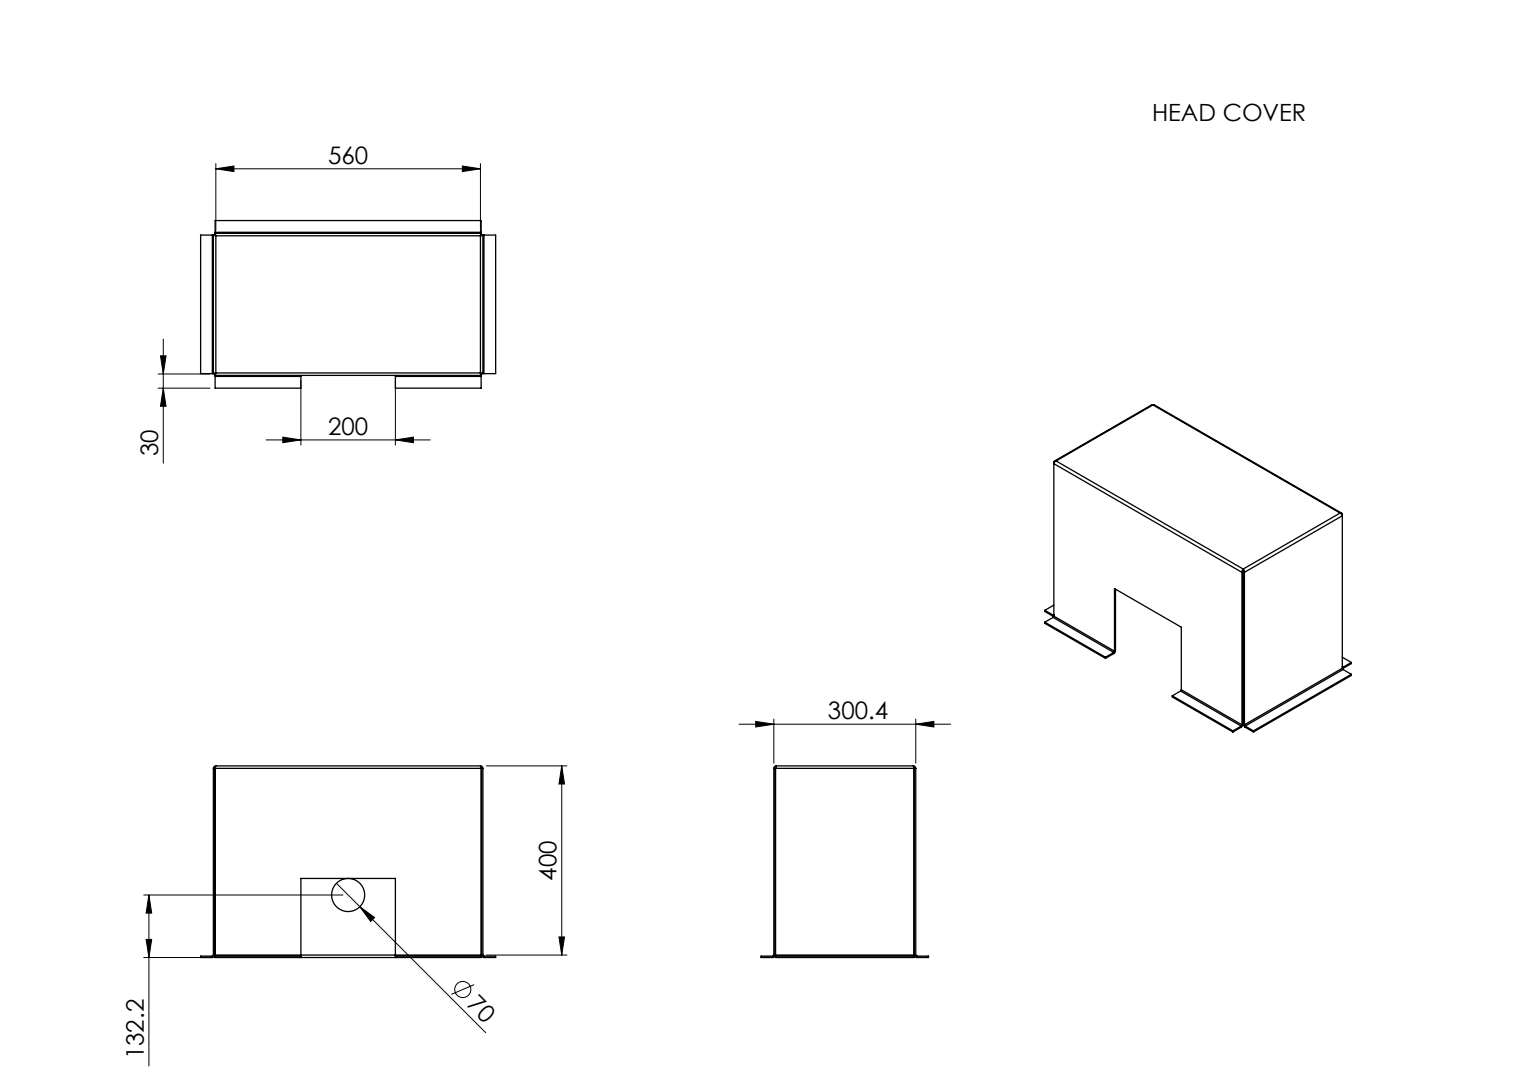
ISO-10303-21;
HEADER;
FILE_DESCRIPTION (('STEP AP214'),
    '1' );
FILE_NAME ('head cover.step',
    '2026-10-31T03:46:07',
    ( '' ),
    ( '' ),
    'SwSTEP 2.0',
    'SolidWorks 2026',
    '' );
FILE_SCHEMA (( 'AUTOMOTIVE_DESIGN' ));
ENDSEC;

DATA;
#14=DIRECTION ( 'NONE',  ( 1.000000000000000000, -6.640089860198304064E-16, -0.000000000000000000 ) ) ;
#17=AXIS2_PLACEMENT_3D ( 'NONE', #8698, #6875, #2876 ) ;
#23=DIRECTION ( 'NONE',  ( -0.000000000000000000, -0.000000000000000000, 1.000000000000000000 ) ) ;
#39=VECTOR ( 'NONE', #3560, 1000.000000000000000 ) ;
#44=CARTESIAN_POINT ( 'NONE',  ( 280.4976310729377929, 269.6958543268122526, -146.0927021017107279 ) ) ;
#46=DIRECTION ( 'NONE',  ( 1.000000000000000000, -0.000000000000000000, -0.000000000000000000 ) ) ;
#47=EDGE_LOOP ( 'NONE', ( #6115, #19407 ) ) ;
#50=CARTESIAN_POINT ( 'NONE',  ( 281.4928932188134354, -129.2000000000000455, -150.2000000000013245 ) ) ;
#59=EDGE_CURVE ( 'NONE', #14664, #1301, #12963, .T. ) ;
#62=EDGE_CURVE ( 'NONE', #22159, #2544, #22076, .T. ) ;
#67=VERTEX_POINT ( 'NONE', #12958 ) ;
#68=CARTESIAN_POINT ( 'NONE',  ( 281.3673618604586295, 268.0905802150185195, -147.1999999999998749 ) ) ;
#84=EDGE_CURVE ( 'NONE', #20571, #4595, #14131, .T. ) ;
#87=DIRECTION ( 'NONE',  ( -1.000000000000000000, -0.000000000000000000, -0.000000000000000000 ) ) ;
#101=ORIENTED_EDGE ( 'NONE', *, *, #6605, .F. ) ;
#117=ADVANCED_FACE ( 'NONE', ( #14863 ), #10660, .T. ) ;
#128=CARTESIAN_POINT ( 'NONE',  ( 281.4928932188134354, -132.2000000000000455, -177.2000000000013529 ) ) ;
#129=AXIS2_PLACEMENT_3D ( 'NONE', #9738, #17091, #22629 ) ;
#131=CARTESIAN_POINT ( 'NONE',  ( 284.6730547946947354, 270.1059783239180661, 146.0571358042176087 ) ) ;
#139=FACE_BOUND ( 'NONE', #47, .T. ) ;
#146=ADVANCED_FACE ( 'NONE', ( #21970 ), #14402, .F. ) ;
#147=ORIENTED_EDGE ( 'NONE', *, *, #7523, .T. ) ;
#167=DIRECTION ( 'NONE',  ( 0.000000000000000000, 0.000000000000000000, -1.000000000000000000 ) ) ;
#168=VECTOR ( 'NONE', #12826, 1000.000000000000000 ) ;
#171=EDGE_CURVE ( 'NONE', #22518, #4872, #9420, .T. ) ;
#177=CARTESIAN_POINT ( 'NONE',  ( -34.75000000000005684, 100.0000000000000000, 150.2000000000009550 ) ) ;
#185=EDGE_CURVE ( 'NONE', #19310, #4045, #11744, .T. ) ;
#202=CIRCLE ( 'NONE', #14864, 2.649999999999971934 ) ;
#210=CARTESIAN_POINT ( 'NONE',  ( 281.1021437883072167, 269.7094021484633686, -145.4974534559949859 ) ) ;
#211=EDGE_LOOP ( 'NONE', ( #6410, #3286, #15490, #21044 ) ) ;
#212=ADVANCED_FACE ( 'NONE', ( #22806 ), #18937, .T. ) ;
#225=VECTOR ( 'NONE', #9857, 1000.000000000000000 ) ;
#231=ORIENTED_EDGE ( 'NONE', *, *, #16834, .F. ) ;
#233=LINE ( 'NONE', #3596, #6438 ) ;
#244=DIRECTION ( 'NONE',  ( 1.000000000000000000, -0.000000000000000000, -0.000000000000000000 ) ) ;
#249=CARTESIAN_POINT ( 'NONE',  ( -100.0000000000000000, 35.00000000000009948, 150.2000000000008413 ) ) ;
#263=DIRECTION ( 'NONE',  ( 1.000000000000000000, 0.000000000000000000, 0.000000000000000000 ) ) ;
#264=ORIENTED_EDGE ( 'NONE', *, *, #1576, .T. ) ;
#265=CARTESIAN_POINT ( 'NONE',  ( 280.3431883566700549, 273.0000000000000568, -145.0627246244601167 ) ) ;
#270=ADVANCED_FACE ( 'NONE', ( #15223 ), #15473, .F. ) ;
#276=ORIENTED_EDGE ( 'NONE', *, *, #12482, .T. ) ;
#284=CARTESIAN_POINT ( 'NONE',  ( -280.9952621458755857, 268.9079617568159506, -146.9223300543793584 ) ) ;
#289=LINE ( 'NONE', #9594, #2999 ) ;
#291=AXIS2_PLACEMENT_3D ( 'NONE', #21240, #8314, #10626 ) ;
#292=CARTESIAN_POINT ( 'NONE',  ( 281.8958543268121844, 268.8927021017106540, 145.9952621458756710 ) ) ;
#297=FACE_OUTER_BOUND ( 'NONE', #16595, .T. ) ;
#313=EDGE_CURVE ( 'NONE', #14070, #15403, #21354, .T. ) ;
#331=VECTOR ( 'NONE', #4440, 1000.000000000000000 ) ;
#336=AXIS2_PLACEMENT_3D ( 'NONE', #12749, #1460, #5215 ) ;
#340=DIRECTION ( 'NONE',  ( -1.000000000000000000, -0.000000000000000000, -0.000000000000000000 ) ) ;
#341=AXIS2_PLACEMENT_3D ( 'NONE', #13845, #16102, #21173 ) ;
#351=ADVANCED_FACE ( 'NONE', ( #21114 ), #3118, .F. ) ;
#352=ORIENTED_EDGE ( 'NONE', *, *, #7831, .T. ) ;
#355=AXIS2_PLACEMENT_3D ( 'NONE', #12926, #14588, #3930 ) ;
#367=DIRECTION ( 'NONE',  ( 1.000000000000000000, 0.000000000000000000, -0.000000000000000000 ) ) ;
#368=EDGE_LOOP ( 'NONE', ( #6453, #4293, #7528, #16012 ) ) ;
#372=AXIS2_PLACEMENT_3D ( 'NONE', #12914, #5396, #21586 ) ;
#381=VECTOR ( 'NONE', #12199, 1000.000000000000000 ) ;
#382=CARTESIAN_POINT ( 'NONE',  ( -280.4973317504632746, 272.3135885331259374, -147.6045710003933493 ) ) ;
#384=CARTESIAN_POINT ( 'NONE',  ( -281.4538215477170979, 269.4574776399289249, -145.6842353883612304 ) ) ;
#386=LINE ( 'NONE', #9552, #2401 ) ;
#396=CARTESIAN_POINT ( 'NONE',  ( 280.4976310729377929, 272.3436892194421830, -147.6188186979286456 ) ) ;
#416=CIRCLE ( 'NONE', #20853, 2.649999999999975486 ) ;
#421=CARTESIAN_POINT ( 'NONE',  ( -280.1244266708878854, 270.0000000000000000, -145.2880230824753198 ) ) ;
#430=EDGE_LOOP ( 'NONE', ( #19662, #7339, #6676, #22145 ) ) ;
#458=ADVANCED_FACE ( 'NONE', ( #6629 ), #8833, .F. ) ;
#459=CARTESIAN_POINT ( 'NONE',  ( 282.1854425596106921, 268.0906609804447953, -146.3673129565597719 ) ) ;
#460=EDGE_CURVE ( 'NONE', #4025, #10987, #14591, .T. ) ;
#472=CARTESIAN_POINT ( 'NONE',  ( 281.9223300543793584, 268.9079617568158938, -145.9952621458755857 ) ) ;
#477=ORIENTED_EDGE ( 'NONE', *, *, #2966, .T. ) ;
#478=ORIENTED_EDGE ( 'NONE', *, *, #11288, .T. ) ;
#481=ADVANCED_FACE ( 'NONE', ( #3691 ), #14484, .T. ) ;
#484=EDGE_LOOP ( 'NONE', ( #635, #3339, #8583, #20621 ) ) ;
#497=CARTESIAN_POINT ( 'NONE',  ( -280.1452901038203436, 270.0000000000000000, -145.0627656775836556 ) ) ;
#500=DIRECTION ( 'NONE',  ( 0.000000000000000000, -3.495664435217746987E-15, -1.000000000000000000 ) ) ;
#502=FACE_BOUND ( 'NONE', #1152, .T. ) ;
#503=DIRECTION ( 'NONE',  ( 0.000000000000000000, 0.000000000000000000, 1.000000000000000000 ) ) ;
#505=VECTOR ( 'NONE', #4591, 1000.000000000000000 ) ;
#515=EDGE_CURVE ( 'NONE', #17412, #8986, #3345, .T. ) ;
#530=CARTESIAN_POINT ( 'NONE',  ( -282.0873946496627127, 268.5095819834011763, 146.1815513148989965 ) ) ;
#539=VERTEX_POINT ( 'NONE', #2242 ) ;
#541=CYLINDRICAL_SURFACE ( 'NONE', #20678, 2.199999999999979750 ) ;
#549=CARTESIAN_POINT ( 'NONE',  ( -280.0000000000000568, 272.9999999999999432, 145.0000000000000284 ) ) ;
#558=EDGE_CURVE ( 'NONE', #7386, #12822, #19852, .T. ) ;
#559=CARTESIAN_POINT ( 'NONE',  ( -288.2000000000013529, -89.99999999999897682, 26.98333333333330231 ) ) ;
#577=EDGE_CURVE ( 'NONE', #539, #10685, #15195, .T. ) ;
#584=FACE_BOUND ( 'NONE', #11064, .T. ) ;
#594=EDGE_CURVE ( 'NONE', #15324, #17025, #2363, .T. ) ;
#603=VERTEX_POINT ( 'NONE', #15316 ) ;
#604=CARTESIAN_POINT ( 'NONE',  ( 285.2000000000008981, 9.892604858775018348E-13, 146.4928932188134638 ) ) ;
#614=CARTESIAN_POINT ( 'NONE',  ( 280.6822561791009889, 272.9663407402829876, 145.1247002395580807 ) ) ;
#617=CARTESIAN_POINT ( 'NONE',  ( 40.00000000000000000, 100.0000000000000000, 150.2000000000009550 ) ) ;
#618=ORIENTED_EDGE ( 'NONE', *, *, #2883, .F. ) ;
#621=SURFACE_SIDE_STYLE ('',( #11763 ) ) ;
#625=DIRECTION ( 'NONE',  ( -0.000000000000000000, -0.000000000000000000, 1.000000000000000000 ) ) ;
#631=CARTESIAN_POINT ( 'NONE',  ( 282.6045710003933777, 272.3135885331259942, -145.4973317504631609 ) ) ;
#632=EDGE_LOOP ( 'NONE', ( #21838, #2466, #15904, #21981 ) ) ;
#635=ORIENTED_EDGE ( 'NONE', *, *, #22905, .T. ) ;
#640=VERTEX_POINT ( 'NONE', #19144 ) ;
#641=CARTESIAN_POINT ( 'NONE',  ( -281.3684665762324926, 268.0840560642351988, -147.1696999999999207 ) ) ;
#662=CARTESIAN_POINT ( 'NONE',  ( -285.2000000000013529, -89.99999999999896261, -40.33333333333332860 ) ) ;
#672=PLANE ( 'NONE',  #1139 ) ;
#674=ORIENTED_EDGE ( 'NONE', *, *, #10081, .T. ) ;
#678=AXIS2_PLACEMENT_3D ( 'NONE', #5455, #7253, #20169 ) ;
#686=DIRECTION ( 'NONE',  ( -1.000000000000000000, 3.495664435217746592E-15, -0.000000000000000000 ) ) ;
#689=FACE_OUTER_BOUND ( 'NONE', #8839, .T. ) ;
#693=ORIENTED_EDGE ( 'NONE', *, *, #16007, .T. ) ;
#697=CARTESIAN_POINT ( 'NONE',  ( -282.2000000000006708, 90.00000000000102318, -32.35000000000004405 ) ) ;
#729=FILL_AREA_STYLE ('',( #3980 ) ) ;
#733=VERTEX_POINT ( 'NONE', #21327 ) ;
#734=EDGE_CURVE ( 'NONE', #21032, #15145, #6249, .T. ) ;
#736=CARTESIAN_POINT ( 'NONE',  ( 0.000000000000000000, -132.2000000000000455, 7.703011046602857601E-15 ) ) ;
#746=VECTOR ( 'NONE', #8115, 1000.000000000000000 ) ;
#749=CARTESIAN_POINT ( 'NONE',  ( -280.4976310729379065, 272.3436892194421262, 147.6188186979287025 ) ) ;
#751=ORIENTED_EDGE ( 'NONE', *, *, #3968, .T. ) ;
#752=ADVANCED_FACE ( 'NONE', ( #913 ), #15562, .F. ) ;
#756=DIRECTION ( 'NONE',  ( 1.000000000000000000, 0.000000000000000000, 0.000000000000000000 ) ) ;
#761=CARTESIAN_POINT ( 'NONE',  ( -280.6220388411722411, 271.9822575857424454, -148.2140793454688037 ) ) ;
#769=LINE ( 'NONE', #1117, #4265 ) ;
#770=CARTESIAN_POINT ( 'NONE',  ( 284.1582675804705218, 270.9956429438695409, 145.8708543776411943 ) ) ;
#775=CARTESIAN_POINT ( 'NONE',  ( 45.00000000000000000, 272.9999999999999432, 5.249999999999973355 ) ) ;
#787=EDGE_CURVE ( 'NONE', #23122, #3613, #19452, .T. ) ;
#813=ORIENTED_EDGE ( 'NONE', *, *, #10441, .T. ) ;
#822=DIRECTION ( 'NONE',  ( 0.000000000000000000, -1.000000000000000000, -3.172065784643303781E-15 ) ) ;
#823=CARTESIAN_POINT ( 'NONE',  ( -280.0000000000000568, 272.9999999999999432, 145.0000000000000284 ) ) ;
#830=ORIENTED_EDGE ( 'NONE', *, *, #12374, .F. ) ;
#838=DIRECTION ( 'NONE',  ( 1.000000000000000000, 0.000000000000000000, -0.000000000000000000 ) ) ;
#845=DIRECTION ( 'NONE',  ( 0.000000000000000000, 0.000000000000000000, -1.000000000000000000 ) ) ;
#851=VECTOR ( 'NONE', #20972, 1000.000000000000000 ) ;
#858=CARTESIAN_POINT ( 'NONE',  ( -281.2440776823446527, 269.1689414351989740, 150.0938770989752982 ) ) ;
#861=ADVANCED_FACE ( 'NONE', ( #22030 ), #21930, .F. ) ;
#862=FACE_BOUND ( 'NONE', #14300, .T. ) ;
#872=EDGE_CURVE ( 'NONE', #15992, #2924, #11012, .T. ) ;
#887=ORIENTED_EDGE ( 'NONE', *, *, #20314, .T. ) ;
#899=CARTESIAN_POINT ( 'NONE',  ( 281.7502846751310699, 269.1405375976306686, 145.8716261326570702 ) ) ;
#905=DIRECTION ( 'NONE',  ( 0.000000000000000000, -1.000000000000000000, 0.000000000000000000 ) ) ;
#913=FACE_OUTER_BOUND ( 'NONE', #11726, .T. ) ;
#933=CARTESIAN_POINT ( 'NONE',  ( 280.2481149223240209, 269.9433523009094529, 145.5743436287470161 ) ) ;
#955=PLANE ( 'NONE',  #7810 ) ;
#967=CARTESIAN_POINT ( 'NONE',  ( 281.4928932188133217, -127.0000000000000568, 152.4000000000014268 ) ) ;
#971=CARTESIAN_POINT ( 'NONE',  ( -281.2440776823446527, 268.3758453455903918, 147.1427398886702917 ) ) ;
#988=CARTESIAN_POINT ( 'NONE',  ( -281.4928932188134922, -127.0000000000000568, -150.2000000000013245 ) ) ;
#990=CARTESIAN_POINT ( 'NONE',  ( -281.4928932188135491, -132.2000000000000455, 177.2000000000014097 ) ) ;
#995=EDGE_CURVE ( 'NONE', #20571, #18758, #14923, .T. ) ;
#1006=VECTOR ( 'NONE', #14424, 1000.000000000000000 ) ;
#1011=CARTESIAN_POINT ( 'NONE',  ( -100.0000000000001137, -129.2000000000000455, 7.690461757479017101E-15 ) ) ;
#1020=ORIENTED_EDGE ( 'NONE', *, *, #23692, .T. ) ;
#1021=CARTESIAN_POINT ( 'NONE',  ( 285.2000000000013529, -129.2000000000000455, 146.4928932188134638 ) ) ;
#1030=ADVANCED_FACE ( 'NONE', ( #12132 ), #13818, .F. ) ;
#1049=CARTESIAN_POINT ( 'NONE',  ( -285.1663407402830899, 268.4822561791010571, 146.3681929792554399 ) ) ;
#1055=ORIENTED_EDGE ( 'NONE', *, *, #2680, .T. ) ;
#1058=ORIENTED_EDGE ( 'NONE', *, *, #22905, .F. ) ;
#1075=EDGE_CURVE ( 'NONE', #603, #2349, #20263, .T. ) ;
#1077=CIRCLE ( 'NONE', #20722, 2.649999999999975486 ) ;
#1087=B_SPLINE_CURVE_WITH_KNOTS ( 'NONE', 3,
 ( #11660, #265, #22590, #2179, #6054, #2428, #631, #20787, #11774, #19083, #2552, #18965, #5699, #16697, #13235, #7624, #22361, #15016, #20427, #4250 ),
 .UNSPECIFIED., .F., .F.,
 ( 4, 2, 2, 2, 2, 2, 2, 2, 2, 4 ),
 ( 0.000000000000000000, 0.001035985217005840064, 0.002071970434011680129, 0.003107955651017520193, 0.003625948259520417674, 0.004143940868023315155, 0.005179926085028993023, 0.006215911302034670891, 0.007251896519040349626, 0.008287881736046026626 ),
 .UNSPECIFIED. ) ;
#1093=B_SPLINE_SURFACE_WITH_KNOTS ( 'NONE', 1, 3, ( 
 ( #5953, #2443, #17190, #3899, #761, #22488, #15389, #11788, #13611, #5842 ),
 ( #8012, #9835, #15273, #22379, #13362, #18733, #9472, #5713, #22605, #11672 ),
 ( #9589, #421, #7890, #13250, #20553, #4129, #284, #17313, #15155, #7774 ),
 ( #20804, #4007, #11424, #15036, #20921, #8143, #20674, #2194, #641, #16953 ) ),
 .UNSPECIFIED., .F., .F., .F.,
 ( 2, 1, 1, 2 ),
 ( 4, 2, 2, 2, 4 ),
 ( -0.01000000000000000021, 0.000000000000000000, 1.000000000000000000, 1.010099999999999998 ),
 ( 0.000000000000000000, 0.2500000000000000000, 0.5000000000000000000, 0.7500000000000000000, 1.000000000000000000 ),
 .UNSPECIFIED. ) ;
#1099=ORIENTED_EDGE ( 'NONE', *, *, #23146, .F. ) ;
#1102=CARTESIAN_POINT ( 'NONE',  ( -281.4928932188135491, 267.7999999999999545, 147.1999999999999886 ) ) ;
#1114=VECTOR ( 'NONE', #12180, 1000.000000000000000 ) ;
#1115=VECTOR ( 'NONE', #10599, 1000.000000000000000 ) ;
#1117=CARTESIAN_POINT ( 'NONE',  ( 35.00000000000000711, 0.000000000000000000, -177.2000000000013529 ) ) ;
#1119=AXIS2_PLACEMENT_3D ( 'NONE', #5628, #14944, #12816 ) ;
#1123=DIRECTION ( 'NONE',  ( -0.000000000000000000, 1.000000000000000000, -4.183096374613631247E-18 ) ) ;
#1124=CARTESIAN_POINT ( 'NONE',  ( -285.0646579186753797, 269.1610889986682196, -146.2440776823445390 ) ) ;
#1128=DIRECTION ( 'NONE',  ( -0.000000000000000000, 0.000000000000000000, -1.000000000000000000 ) ) ;
#1130=ADVANCED_FACE ( 'NONE', ( #17882 ), #23560, .F. ) ;
#1139=AXIS2_PLACEMENT_3D ( 'NONE', #8048, #21315, #12297 ) ;
#1147=CARTESIAN_POINT ( 'NONE',  ( 280.9755403010747159, 269.7771302778489826, 145.4357197208657340 ) ) ;
#1152=EDGE_LOOP ( 'NONE', ( #4727, #12791 ) ) ;
#1162=CIRCLE ( 'NONE', #12782, 2.199999999999979750 ) ;
#1164=CARTESIAN_POINT ( 'NONE',  ( -281.4928932188135491, -132.2000000000000455, 150.2000000000013813 ) ) ;
#1167=CARTESIAN_POINT ( 'NONE',  ( -283.7968359015655437, 271.3570580646226631, -145.7774350431394907 ) ) ;
#1174=DIRECTION ( 'NONE',  ( 0.000000000000000000, 0.000000000000000000, 1.000000000000000000 ) ) ;
#1176=DIRECTION ( 'NONE',  ( 4.183096374613631247E-18, -1.000000000000000000, 0.000000000000000000 ) ) ;
#1183=VECTOR ( 'NONE', #18740, 1000.000000000000000 ) ;
#1185=ORIENTED_EDGE ( 'NONE', *, *, #3808, .F. ) ;
#1186=CARTESIAN_POINT ( 'NONE',  ( -281.2431816561011715, 268.3724317483737423, -147.1290760626066856 ) ) ;
#1203=ORIENTED_EDGE ( 'NONE', *, *, #19391, .F. ) ;
#1211=ORIENTED_EDGE ( 'NONE', *, *, #5766, .T. ) ;
#1213=DIRECTION ( 'NONE',  ( -0.000000000000000000, 7.709882115452476934E-17, -1.000000000000000000 ) ) ;
#1216=VERTEX_POINT ( 'NONE', #21849 ) ;
#1221=EDGE_CURVE ( 'NONE', #21906, #11842, #4475, .T. ) ;
#1224=ORIENTED_EDGE ( 'NONE', *, *, #9825, .T. ) ;
#1226=CARTESIAN_POINT ( 'NONE',  ( 0.000000000000000000, 5.173457871231059415E-13, -150.2000000000008981 ) ) ;
#1227=FACE_OUTER_BOUND ( 'NONE', #1740, .T. ) ;
#1238=DIRECTION ( 'NONE',  ( -0.000000000000000000, 0.000000000000000000, 1.000000000000000000 ) ) ;
#1274=CARTESIAN_POINT ( 'NONE',  ( -284.2295083325149108, 270.8299054689546779, -145.9020829022173871 ) ) ;
#1284=VECTOR ( 'NONE', #5986, 1000.000000000000000 ) ;
#1285=CARTESIAN_POINT ( 'NONE',  ( 281.4928932188133786, -129.2000000000000455, 177.2000000000014097 ) ) ;
#1289=DIRECTION ( 'NONE',  ( 4.183096374613631247E-18, 1.000000000000000000, 0.000000000000000000 ) ) ;
#1291=ORIENTED_EDGE ( 'NONE', *, *, #17411, .F. ) ;
#1293=LINE ( 'NONE', #1412, #19171 ) ;
#1301=VERTEX_POINT ( 'NONE', #22323 ) ;
#1303=ADVANCED_FACE ( 'NONE', ( #4461 ), #20888, .F. ) ;
#1308=ORIENTED_EDGE ( 'NONE', *, *, #15523, .F. ) ;
#1320=CARTESIAN_POINT ( 'NONE',  ( -312.2000000000014666, -132.2000000000000455, -146.4928932188134070 ) ) ;
#1321=EDGE_CURVE ( 'NONE', #13384, #21062, #15345, .T. ) ;
#1330=ORIENTED_EDGE ( 'NONE', *, *, #4417, .T. ) ;
#1342=DIRECTION ( 'NONE',  ( 1.000000000000000000, -6.938893903907227392E-16, 0.000000000000000000 ) ) ;
#1343=DIRECTION ( 'NONE',  ( 0.000000000000000000, 0.000000000000000000, -1.000000000000000000 ) ) ;
#1347=DIRECTION ( 'NONE',  ( 0.000000000000000000, 1.000000000000000000, -5.286776307738891306E-15 ) ) ;
#1350=EDGE_CURVE ( 'NONE', #9824, #17073, #13684, .T. ) ;
#1356=CARTESIAN_POINT ( 'NONE',  ( -288.2000000000006708, 90.00000000000100897, 34.99999999999999289 ) ) ;
#1359=CIRCLE ( 'NONE', #4052, 5.199999999999982414 ) ;
#1360=ORIENTED_EDGE ( 'NONE', *, *, #12442, .T. ) ;
#1370=CARTESIAN_POINT ( 'NONE',  ( 282.1999999999999318, 267.7999999999999545, 146.4928932188134922 ) ) ;
#1378=VECTOR ( 'NONE', #2350, 1000.000000000000000 ) ;
#1412=CARTESIAN_POINT ( 'NONE',  ( -281.4928932188135491, -129.2000000000000455, 177.2000000000014097 ) ) ;
#1415=CARTESIAN_POINT ( 'NONE',  ( 284.1822575857424340, 271.0140793454687582, -145.8708543776411091 ) ) ;
#1427=DIRECTION ( 'NONE',  ( 0.000000000000000000, 0.000000000000000000, -1.000000000000000000 ) ) ;
#1429=ORIENTED_EDGE ( 'NONE', *, *, #12122, .F. ) ;
#1430=EDGE_CURVE ( 'NONE', #14150, #10594, #202, .T. ) ;
#1445=CARTESIAN_POINT ( 'NONE',  ( 0.000000000000000000, -129.2000000000000455, -7.690461757479017101E-15 ) ) ;
#1453=EDGE_LOOP ( 'NONE', ( #17995, #9504, #17274, #20589 ) ) ;
#1458=CARTESIAN_POINT ( 'NONE',  ( -100.0000000000001137, -132.2000000000001592, 177.2000000000014097 ) ) ;
#1460=DIRECTION ( 'NONE',  ( 0.000000000000000000, -4.183096374613631247E-18, -1.000000000000000000 ) ) ;
#1469=PLANE ( 'NONE',  #22255 ) ;
#1484=VECTOR ( 'NONE', #21691, 1000.000000000000000 ) ;
#1497=CARTESIAN_POINT ( 'NONE',  ( -45.00000000000000000, 269.9999999999999432, -5.249999999999973355 ) ) ;
#1505=APPLICATION_CONTEXT ( 'automotive_design' ) ;
#1507=CARTESIAN_POINT ( 'NONE',  ( -281.4928932188134354, -129.2000000000000455, -152.4000000000012562 ) ) ;
#1516=EDGE_CURVE ( 'NONE', #9258, #16083, #23169, .T. ) ;
#1519=AXIS2_PLACEMENT_3D ( 'NONE', #4350, #20765, #2163 ) ;
#1525=LINE ( 'NONE', #7427, #20637 ) ;
#1530=CARTESIAN_POINT ( 'NONE',  ( 287.4000000000013415, -132.2000000000000455, 146.4928932188134638 ) ) ;
#1531=CYLINDRICAL_SURFACE ( 'NONE', #372, 2.649999999999971934 ) ;
#1534=CARTESIAN_POINT ( 'NONE',  ( -312.2000000000014666, -132.2000000000000455, 146.4928932188134638 ) ) ;
#1536=ORIENTED_EDGE ( 'NONE', *, *, #16790, .F. ) ;
#1537=ORIENTED_EDGE ( 'NONE', *, *, #7567, .T. ) ;
#1550=CARTESIAN_POINT ( 'NONE',  ( 281.4928932188133217, 267.7999999999999545, 150.1999999999999886 ) ) ;
#1553=EDGE_LOOP ( 'NONE', ( #17397, #4963, #19044, #3864 ) ) ;
#1564=CARTESIAN_POINT ( 'NONE',  ( 284.5436892194421148, 270.4188186979286002, -145.9952621458755857 ) ) ;
#1576=EDGE_CURVE ( 'NONE', #22418, #12831, #6749, .T. ) ;
#1585=CARTESIAN_POINT ( 'NONE',  ( -280.1255802622537203, 269.9854425596105898, 145.2906609804448124 ) ) ;
#1587=DIRECTION ( 'NONE',  ( 0.000000000000000000, 0.000000000000000000, 1.000000000000000000 ) ) ;
#1599=LINE ( 'NONE', #12992, #15732 ) ;
#1619=CARTESIAN_POINT ( 'NONE',  ( 40.00000000000000000, 100.0000000000000000, 150.2000000000009550 ) ) ;
#1622=DIRECTION ( 'NONE',  ( 0.000000000000000000, 1.000000000000000000, -0.000000000000000000 ) ) ;
#1625=CARTESIAN_POINT ( 'NONE',  ( -285.2300000000000182, 267.7999999999999545, 146.4928932188134354 ) ) ;
#1627=CARTESIAN_POINT ( 'NONE',  ( 280.8083875057488967, 271.2314821058791949, -148.9107452280323116 ) ) ;
#1640=LINE ( 'NONE', #21917, #39 ) ;
#1643=LINE ( 'NONE', #3459, #13493 ) ;
#1647=VERTEX_POINT ( 'NONE', #6995 ) ;
#1651=FACE_OUTER_BOUND ( 'NONE', #10746, .T. ) ;
#1653=ORIENTED_EDGE ( 'NONE', *, *, #17686, .F. ) ;
#1657=CARTESIAN_POINT ( 'NONE',  ( 280.1244266425809428, 269.9696999999999889, 145.2840560642353580 ) ) ;
#1665=FACE_OUTER_BOUND ( 'NONE', #16076, .T. ) ;
#1670=CARTESIAN_POINT ( 'NONE',  ( 284.5699028110927316, 270.4339272673396977, -145.9952621458755857 ) ) ;
#1674=VECTOR ( 'NONE', #9828, 1000.000000000000000 ) ;
#1701=VECTOR ( 'NONE', #22770, 1000.000000000000000 ) ;
#1714=CARTESIAN_POINT ( 'NONE',  ( -282.2000000000013529, -89.99999999999896261, -40.33333333333332860 ) ) ;
#1718=AXIS2_PLACEMENT_3D ( 'NONE', #14058, #10435, #15617 ) ;
#1719=DIRECTION ( 'NONE',  ( -0.000000000000000000, -0.000000000000000000, 1.000000000000000000 ) ) ;
#1734=CARTESIAN_POINT ( 'NONE',  ( -284.1822575857425477, 271.0140793454687582, 145.8708543776411659 ) ) ;
#1740=EDGE_LOOP ( 'NONE', ( #20447, #18390, #7293, #13753 ) ) ;
#1755=DIRECTION ( 'NONE',  ( 0.000000000000000000, -3.495664435217746987E-15, -1.000000000000000000 ) ) ;
#1765=EDGE_CURVE ( 'NONE', #16905, #21880, #22652, .T. ) ;
#1767=ORIENTED_EDGE ( 'NONE', *, *, #15455, .F. ) ;
#1768=DIRECTION ( 'NONE',  ( 0.000000000000000000, -1.000000000000000000, -3.172065784643303781E-15 ) ) ;
#1772=ORIENTED_EDGE ( 'NONE', *, *, #17021, .F. ) ;
#1778=ORIENTED_EDGE ( 'NONE', *, *, #7984, .T. ) ;
#1798=ADVANCED_FACE ( 'NONE', ( #16753 ), #11465, .F. ) ;
#1804=PLANE ( 'NONE',  #15058 ) ;
#1806=PLANE ( 'NONE',  #4570 ) ;
#1814=( LENGTH_UNIT ( ) NAMED_UNIT ( * ) SI_UNIT ( .MILLI., .METRE. ) );
#1820=CARTESIAN_POINT ( 'NONE',  ( 280.1244266425809428, 269.9697000000000457, -145.2840560642351875 ) ) ;
#1848=CARTESIAN_POINT ( 'NONE',  ( -282.2000000000008981, 35.00000000000100897, 105.0000000000000000 ) ) ;
#1852=DIRECTION ( 'NONE',  ( -0.000000000000000000, -0.000000000000000000, 1.000000000000000000 ) ) ;
#1869=CARTESIAN_POINT ( 'NONE',  ( -281.4928932188134354, -129.2000000000000455, -177.2000000000013529 ) ) ;
#1873=LINE ( 'NONE', #22157, #4371 ) ;
#1874=ORIENTED_EDGE ( 'NONE', *, *, #16107, .F. ) ;
#1885=AXIS2_PLACEMENT_3D ( 'NONE', #1848, #5137, #12796 ) ;
#1886=CARTESIAN_POINT ( 'NONE',  ( 279.9999999999999432, 269.9999999999999432, 145.0000000000000284 ) ) ;
#1887=VECTOR ( 'NONE', #1959, 1000.000000000000000 ) ;
#1896=DIRECTION ( 'NONE',  ( 0.000000000000000000, -1.000000000000000000, 0.000000000000000000 ) ) ;
#1924=( GEOMETRIC_REPRESENTATION_CONTEXT ( 3 ) GLOBAL_UNCERTAINTY_ASSIGNED_CONTEXT ( ( #2665 ) ) GLOBAL_UNIT_ASSIGNED_CONTEXT ( ( #1814, #2662, #15492 ) ) REPRESENTATION_CONTEXT ( 'NONE', 'WORKASPACE' ) );
#1925=AXIS2_PLACEMENT_3D ( 'NONE', #11459, #17111, #17003 ) ;
#1926=CIRCLE ( 'NONE', #15467, 2.199999999999979750 ) ;
#1936=CARTESIAN_POINT ( 'NONE',  ( -282.2000000000000455, 267.7999999999999545, -146.4928932188134354 ) ) ;
#1938=CARTESIAN_POINT ( 'NONE',  ( 99.99999999999987210, -127.0000000000000853, 147.2000000000013529 ) ) ;
#1948=ADVANCED_FACE ( 'NONE', ( #5038 ), #3192, .F. ) ;
#1950=DIRECTION ( 'NONE',  ( -0.000000000000000000, -0.000000000000000000, 1.000000000000000000 ) ) ;
#1959=DIRECTION ( 'NONE',  ( -0.000000000000000000, -0.000000000000000000, 1.000000000000000000 ) ) ;
#1972=EDGE_CURVE ( 'NONE', #19310, #20612, #19745, .T. ) ;
#1973=DIRECTION ( 'NONE',  ( 0.000000000000000000, -3.491481338843133355E-15, -1.000000000000000000 ) ) ;
#1974=LINE ( 'NONE', #2088, #1183 ) ;
#1979=LINE ( 'NONE', #16836, #16431 ) ;
#1981=DIRECTION ( 'NONE',  ( 0.000000000000000000, -0.000000000000000000, 1.000000000000000000 ) ) ;
#1983=ORIENTED_EDGE ( 'NONE', *, *, #11069, .T. ) ;
#1988=ORIENTED_EDGE ( 'NONE', *, *, #19088, .F. ) ;
#1992=DIRECTION ( 'NONE',  ( 0.000000000000000000, -1.000000000000000000, -5.286776307738891306E-15 ) ) ;
#1999=LINE ( 'NONE', #18545, #5388 ) ;
#2011=DIRECTION ( 'NONE',  ( 0.000000000000000000, -1.000000000000000000, 0.000000000000000000 ) ) ;
#2022=DIRECTION ( 'NONE',  ( -1.000000000000000000, 3.495664435217746987E-15, 0.000000000000000000 ) ) ;
#2025=EDGE_CURVE ( 'NONE', #22322, #15324, #12552, .T. ) ;
#2028=DIRECTION ( 'NONE',  ( 0.000000000000000000, 0.000000000000000000, 1.000000000000000000 ) ) ;
#2029=FACE_OUTER_BOUND ( 'NONE', #11694, .T. ) ;
#2039=VECTOR ( 'NONE', #10467, 1000.000000000000000 ) ;
#2040=ADVANCED_FACE ( 'NONE', ( #23719 ), #16138, .T. ) ;
#2041=FACE_OUTER_BOUND ( 'NONE', #5191, .T. ) ;
#2044=VECTOR ( 'NONE', #18359, 1000.000000000000000 ) ;
#2047=EDGE_LOOP ( 'NONE', ( #14884, #22108, #1224, #7071 ) ) ;
#2055=CARTESIAN_POINT ( 'NONE',  ( 45.24999999999994316, 100.0000000000000000, 150.2000000000009550 ) ) ;
#2056=ORIENTED_EDGE ( 'NONE', *, *, #3809, .T. ) ;
#2063=ADVANCED_FACE ( 'NONE', ( #297 ), #541, .F. ) ;
#2085=ORIENTED_EDGE ( 'NONE', *, *, #460, .T. ) ;
#2088=CARTESIAN_POINT ( 'NONE',  ( -282.2000000000007276, 75.00000000000099476, -90.00000000000000000 ) ) ;
#2095=EDGE_LOOP ( 'NONE', ( #19025, #1291, #11024, #6887 ) ) ;
#2097=ORIENTED_EDGE ( 'NONE', *, *, #6210, .F. ) ;
#2104=ORIENTED_EDGE ( 'NONE', *, *, #19525, .F. ) ;
#2107=DIRECTION ( 'NONE',  ( -0.000000000000000000, -1.000000000000000000, 3.495664435217746987E-15 ) ) ;
#2112=VECTOR ( 'NONE', #4939, 1000.000000000000000 ) ;
#2123=ORIENTED_EDGE ( 'NONE', *, *, #21274, .F. ) ;
#2134=AXIS2_PLACEMENT_3D ( 'NONE', #1714, #20186, #5705 ) ;
#2136=CARTESIAN_POINT ( 'NONE',  ( -285.2000000000010118, 9.892604858775022387E-13, 0.000000000000000000 ) ) ;
#2141=DIRECTION ( 'NONE',  ( 0.000000000000000000, 0.000000000000000000, 1.000000000000000000 ) ) ;
#2143=DIRECTION ( 'NONE',  ( -0.000000000000000000, -0.000000000000000000, 1.000000000000000000 ) ) ;
#2147=VERTEX_POINT ( 'NONE', #4281 ) ;
#2158=CARTESIAN_POINT ( 'NONE',  ( -280.4357574145959120, 272.4730547946946331, -147.3059783239180547 ) ) ;
#2163=DIRECTION ( 'NONE',  ( -1.000000000000000000, 0.000000000000000000, -0.000000000000000000 ) ) ;
#2171=VERTEX_POINT ( 'NONE', #2211 ) ;
#2172=ORIENTED_EDGE ( 'NONE', *, *, #16834, .T. ) ;
#2175=CARTESIAN_POINT ( 'NONE',  ( 280.8708543776411943, 271.0140793454688151, -149.1822575857424056 ) ) ;
#2179=CARTESIAN_POINT ( 'NONE',  ( 281.3488036478620415, 272.8335297745772436, -145.2489140339769449 ) ) ;
#2180=VERTEX_POINT ( 'NONE', #18526 ) ;
#2182=CARTESIAN_POINT ( 'NONE',  ( -100.0000000000001137, -132.1999999999999602, 152.4000000000014268 ) ) ;
#2194=CARTESIAN_POINT ( 'NONE',  ( -281.2440776823445390, 268.3679143846943589, -147.1132285165672045 ) ) ;
#2197=ADVANCED_FACE ( 'NONE', ( #4147 ), #11560, .F. ) ;
#2198=ORIENTED_EDGE ( 'NONE', *, *, #16661, .T. ) ;
#2200=FACE_OUTER_BOUND ( 'NONE', #20512, .T. ) ;
#2207=ORIENTED_EDGE ( 'NONE', *, *, #5582, .T. ) ;
#2210=CARTESIAN_POINT ( 'NONE',  ( -281.4928932188134922, 5.173457871231059415E-13, -150.2000000000008981 ) ) ;
#2211=CARTESIAN_POINT ( 'NONE',  ( -282.2000000000006708, 90.00000000000102318, -37.64999999999999147 ) ) ;
#2216=CARTESIAN_POINT ( 'NONE',  ( -282.2000000000007276, 75.00000000000099476, -90.00000000000000000 ) ) ;
#2226=AXIS2_PLACEMENT_3D ( 'NONE', #21390, #8489, #4732 ) ;
#2234=CARTESIAN_POINT ( 'NONE',  ( -34.75000000000003553, 100.0000000000000000, 150.2000000000009550 ) ) ;
#2236=ORIENTED_EDGE ( 'NONE', *, *, #17314, .F. ) ;
#2242=CARTESIAN_POINT ( 'NONE',  ( -285.2000000000000455, 267.7999999999999545, 146.4928932188134354 ) ) ;
#2245=AXIS2_PLACEMENT_3D ( 'NONE', #14370, #21589, #20895 ) ;
#2249=CARTESIAN_POINT ( 'NONE',  ( -285.2000000000010687, -19.99999999999898392, 102.3500000000000227 ) ) ;
#2251=CARTESIAN_POINT ( 'NONE',  ( 281.4928932188133217, 267.7999999999999545, 150.1999999999999886 ) ) ;
#2256=SHAPE_DEFINITION_REPRESENTATION ( #7091, #9771 ) ;
#2262=VERTEX_POINT ( 'NONE', #23100 ) ;
#2269=CIRCLE ( 'NONE', #4207, 5.249999999999949374 ) ;
#2278=ORIENTED_EDGE ( 'NONE', *, *, #7743, .F. ) ;
#2287=AXIS2_PLACEMENT_3D ( 'NONE', #23603, #7418, #3311 ) ;
#2288=EDGE_LOOP ( 'NONE', ( #8770, #2316, #14048, #18273 ) ) ;
#2295=CARTESIAN_POINT ( 'NONE',  ( -280.2906609804449545, 269.9854425596107603, -145.1255802622536351 ) ) ;
#2298=CARTESIAN_POINT ( 'NONE',  ( -7.703011046602857601E-15, -132.2000000000000455, -146.4928932188134070 ) ) ;
#2299=ORIENTED_EDGE ( 'NONE', *, *, #7009, .F. ) ;
#2302=ADVANCED_FACE ( 'NONE', ( #11927 ), #6217, .F. ) ;
#2304=EDGE_CURVE ( 'NONE', #22539, #22426, #16759, .T. ) ;
#2308=CARTESIAN_POINT ( 'NONE',  ( 280.9952621458755857, 270.4339272673397545, -149.5699028110927316 ) ) ;
#2309=VECTOR ( 'NONE', #4239, 1000.000000000000000 ) ;
#2310=ORIENTED_EDGE ( 'NONE', *, *, #6574, .F. ) ;
#2311=EDGE_CURVE ( 'NONE', #2349, #5795, #6442, .T. ) ;
#2313=ORIENTED_EDGE ( 'NONE', *, *, #19119, .T. ) ;
#2316=ORIENTED_EDGE ( 'NONE', *, *, #13829, .T. ) ;
#2330=CARTESIAN_POINT ( 'NONE',  ( -281.3405375976307710, 269.5502846751311949, 145.6212670861564504 ) ) ;
#2331=ORIENTED_EDGE ( 'NONE', *, *, #11366, .F. ) ;
#2343=DIRECTION ( 'NONE',  ( 1.000000000000000000, 0.000000000000000000, 0.000000000000000000 ) ) ;
#2349=VERTEX_POINT ( 'NONE', #8027 ) ;
#2350=DIRECTION ( 'NONE',  ( -0.000000000000000000, -0.000000000000000000, 1.000000000000000000 ) ) ;
#2352=ORIENTED_EDGE ( 'NONE', *, *, #2304, .F. ) ;
#2353=CYLINDRICAL_SURFACE ( 'NONE', #129, 2.649999999999971934 ) ;
#2363=B_SPLINE_CURVE_WITH_KNOTS ( 'NONE', 3,
 ( #13285, #22170, #20352, #7446, #210, #11598, #7933, #9645, #11713, #17005, #16643, #20483, #2371, #459, #22287, #3820 ),
 .UNSPECIFIED., .F., .F.,
 ( 4, 2, 2, 2, 2, 2, 2, 4 ),
 ( 0.000000000000000000, 0.0009361184303670160023, 0.001404177645550564986, 0.001872236860734113970, 0.002340296075917663171, 0.002808355291101211938, 0.003276414506284760705, 0.003744473721468309473 ),
 .UNSPECIFIED. ) ;
#2364=ORIENTED_EDGE ( 'NONE', *, *, #8610, .T. ) ;
#2365=CARTESIAN_POINT ( 'NONE',  ( -285.2000000000008981, 35.00000000000100897, 107.6499999999999631 ) ) ;
#2371=CARTESIAN_POINT ( 'NONE',  ( 282.1290760626065435, 268.3724317483735717, -146.2431816561008873 ) ) ;
#2380=CARTESIAN_POINT ( 'NONE',  ( 280.5908103165959346, 272.0295083325147516, 148.0299054689547233 ) ) ;
#2392=ORIENTED_EDGE ( 'NONE', *, *, #171, .F. ) ;
#2394=DIRECTION ( 'NONE',  ( 1.000000000000000000, 0.000000000000000000, 0.000000000000000000 ) ) ;
#2401=VECTOR ( 'NONE', #13328, 1000.000000000000000 ) ;
#2412=CARTESIAN_POINT ( 'NONE',  ( 281.3518577254345132, 272.8327955282140920, 145.2494876630256329 ) ) ;
#2415=PLANE ( 'NONE',  #11196 ) ;
#2421=EDGE_LOOP ( 'NONE', ( #2392, #21606, #2207, #2056 ) ) ;
#2428=CARTESIAN_POINT ( 'NONE',  ( 282.3059783239181115, 272.4730547946948604, -145.4357574145958552 ) ) ;
#2431=CARTESIAN_POINT ( 'NONE',  ( -280.0000000000000568, 269.9999999999999432, 145.0000000000000284 ) ) ;
#2442=ORIENTED_EDGE ( 'NONE', *, *, #21402, .T. ) ;
#2443=CARTESIAN_POINT ( 'NONE',  ( -280.1244295015775378, 273.0299999999999727, -145.6847249064867924 ) ) ;
#2451=CARTESIAN_POINT ( 'NONE',  ( 285.2299999999999045, 268.4847249064869743, 146.3684637172358975 ) ) ;
#2453=ORIENTED_EDGE ( 'NONE', *, *, #12890, .F. ) ;
#2460=CIRCLE ( 'NONE', #5551, 2.649999999999978595 ) ;
#2463=FACE_OUTER_BOUND ( 'NONE', #368, .T. ) ;
#2466=ORIENTED_EDGE ( 'NONE', *, *, #13498, .T. ) ;
#2468=ORIENTED_EDGE ( 'NONE', *, *, #22574, .F. ) ;
#2470=CYLINDRICAL_SURFACE ( 'NONE', #23083, 35.00000000000000711 ) ;
#2473=CARTESIAN_POINT ( 'NONE',  ( -312.2000000000014666, -132.2000000000000455, 0.000000000000000000 ) ) ;
#2489=CARTESIAN_POINT ( 'NONE',  ( -280.0000000000000568, 272.9999999999999432, -144.9999999999999716 ) ) ;
#2503=DIRECTION ( 'NONE',  ( -1.000000000000000000, 3.495664435217746987E-15, 0.000000000000000000 ) ) ;
#2506=CIRCLE ( 'NONE', #1718, 2.649999999999971934 ) ;
#2512=FACE_OUTER_BOUND ( 'NONE', #9395, .T. ) ;
#2516=ORIENTED_EDGE ( 'NONE', *, *, #558, .T. ) ;
#2517=DIRECTION ( 'NONE',  ( 0.000000000000000000, 0.000000000000000000, -1.000000000000000000 ) ) ;
#2544=VERTEX_POINT ( 'NONE', #20541 ) ;
#2547=EDGE_CURVE ( 'NONE', #19084, #13384, #18503, .T. ) ;
#2549=VECTOR ( 'NONE', #11554, 1000.000000000000000 ) ;
#2552=CARTESIAN_POINT ( 'NONE',  ( 283.5570580646225949, 271.5968359015655551, -145.7154581756739162 ) ) ;
#2554=CARTESIAN_POINT ( 'NONE',  ( -280.4976310729379065, 272.3699028110927429, 147.6339272673398284 ) ) ;
#2558=CARTESIAN_POINT ( 'NONE',  ( -281.4928932188135491, 267.7999999999999545, 147.1999999999999886 ) ) ;
#2569=CARTESIAN_POINT ( 'NONE',  ( 285.0646579186752660, 269.1610889986682196, 146.2440776823445958 ) ) ;
#2570=CARTESIAN_POINT ( 'NONE',  ( -282.2000000000000455, 267.7999999999999545, -146.4928932188134354 ) ) ;
#2571=EDGE_CURVE ( 'NONE', #12463, #19820, #7626, .T. ) ;
#2576=VECTOR ( 'NONE', #19776, 1000.000000000000000 ) ;
#2578=DIRECTION ( 'NONE',  ( -1.000000000000000000, 0.000000000000000000, 0.000000000000000000 ) ) ;
#2588=FACE_OUTER_BOUND ( 'NONE', #5104, .T. ) ;
#2589=DIRECTION ( 'NONE',  ( 6.640089860198304064E-16, 1.000000000000000000, -4.183096374613631247E-18 ) ) ;
#2602=ORIENTED_EDGE ( 'NONE', *, *, #17978, .T. ) ;
#2606=DIRECTION ( 'NONE',  ( 1.000000000000000000, 0.000000000000000000, -0.000000000000000000 ) ) ;
#2615=EDGE_CURVE ( 'NONE', #9524, #14070, #7508, .T. ) ;
#2618=ORIENTED_EDGE ( 'NONE', *, *, #20520, .F. ) ;
#2619=CARTESIAN_POINT ( 'NONE',  ( 281.8958543268121844, 268.8927021017106540, -145.9952621458755857 ) ) ;
#2631=VECTOR ( 'NONE', #3825, 1000.000000000000000 ) ;
#2641=ORIENTED_EDGE ( 'NONE', *, *, #12655, .F. ) ;
#2643=EDGE_CURVE ( 'NONE', #20268, #22534, #20021, .T. ) ;
#2650=CARTESIAN_POINT ( 'NONE',  ( -281.4301685938042965, 268.1431883596741841, -150.1999999999999318 ) ) ;
#2651=MECHANICAL_DESIGN_GEOMETRIC_PRESENTATION_REPRESENTATION('',(#5739),#8063);
#2657=VECTOR ( 'NONE', #10679, 1000.000000000000000 ) ;
#2662=( NAMED_UNIT ( * ) PLANE_ANGLE_UNIT ( ) SI_UNIT ( $, .RADIAN. ) );
#2665=UNCERTAINTY_MEASURE_WITH_UNIT (LENGTH_MEASURE( 1.000000000000000082E-05 ), #1814, 'distance_accuracy_value', 'NONE');
#2671=ORIENTED_EDGE ( 'NONE', *, *, #11106, .T. ) ;
#2677=CIRCLE ( 'NONE', #11966, 2.649999999999978595 ) ;
#2680=EDGE_CURVE ( 'NONE', #18466, #16256, #14646, .T. ) ;
#2689=CARTESIAN_POINT ( 'NONE',  ( -282.2000000000012960, -74.99999999999899103, -90.00000000000000000 ) ) ;
#2692=VERTEX_POINT ( 'NONE', #20912 ) ;
#2706=CARTESIAN_POINT ( 'NONE',  ( -285.2000000000000455, 268.4807971656550194, -146.3684637452624884 ) ) ;
#2719=DIRECTION ( 'NONE',  ( 0.000000000000000000, -1.000000000000000000, 0.000000000000000000 ) ) ;
#2726=CARTESIAN_POINT ( 'NONE',  ( 281.9771650631952866, 268.7755899421579784, 146.0571594757292928 ) ) ;
#2727=ADVANCED_FACE ( 'NONE', ( #13956 ), #18089, .F. ) ;
#2749=LINE ( 'NONE', #10135, #18878 ) ;
#2753=CARTESIAN_POINT ( 'NONE',  ( -282.3059783239183389, 272.4730547946946899, 145.4357574145959120 ) ) ;
#2759=ORIENTED_EDGE ( 'NONE', *, *, #7009, .T. ) ;
#2779=VERTEX_POINT ( 'NONE', #18322 ) ;
#2781=VECTOR ( 'NONE', #686, 1000.000000000000000 ) ;
#2784=ORIENTED_EDGE ( 'NONE', *, *, #5582, .F. ) ;
#2787=ORIENTED_EDGE ( 'NONE', *, *, #8816, .F. ) ;
#2788=CARTESIAN_POINT ( 'NONE',  ( -280.8708543776413080, 269.1520027839447948, 146.7592670532760053 ) ) ;
#2791=CARTESIAN_POINT ( 'NONE',  ( -285.2000000000007276, 75.00000000000100897, -90.00000000000000000 ) ) ;
#2792=DIRECTION ( 'NONE',  ( 0.000000000000000000, 1.000000000000000000, 0.000000000000000000 ) ) ;
#2796=ORIENTED_EDGE ( 'NONE', *, *, #6247, .F. ) ;
#2808=CARTESIAN_POINT ( 'NONE',  ( -281.8958543268122980, 268.8927021017106540, -145.9952621458756141 ) ) ;
#2810=AXIS2_PLACEMENT_3D ( 'NONE', #15660, #12299, #2939 ) ;
#2811=CARTESIAN_POINT ( 'NONE',  ( 281.4928932188133217, 267.7999999999999545, 150.1999999999999886 ) ) ;
#2812=EDGE_CURVE ( 'NONE', #15145, #11487, #7202, .T. ) ;
#2813=PRODUCT_DEFINITION ( 'UNKNOWN', '', #9676, #9534 ) ;
#2815=EDGE_CURVE ( 'NONE', #2924, #15992, #8977, .T. ) ;
#2821=ORIENTED_EDGE ( 'NONE', *, *, #12730, .T. ) ;
#2830=ORIENTED_EDGE ( 'NONE', *, *, #1765, .F. ) ;
#2839=EDGE_CURVE ( 'NONE', #12831, #22418, #21921, .T. ) ;
#2842=CYLINDRICAL_SURFACE ( 'NONE', #16942, 2.649999999999971934 ) ;
#2849=LINE ( 'NONE', #1285, #18056 ) ;
#2853=CARTESIAN_POINT ( 'NONE',  ( -281.3488036478622121, 272.8335297745773005, 145.2489140339770017 ) ) ;
#2860=ORIENTED_EDGE ( 'NONE', *, *, #10775, .F. ) ;
#2868=CIRCLE ( 'NONE', #5966, 5.249999999999949374 ) ;
#2870=PLANE ( 'NONE',  #21741 ) ;
#2876=DIRECTION ( 'NONE',  ( 1.000000000000000000, 0.000000000000000000, 0.000000000000000000 ) ) ;
#2883=EDGE_CURVE ( 'NONE', #11842, #20612, #7944, .T. ) ;
#2888=DIRECTION ( 'NONE',  ( 0.000000000000000000, 1.000000000000000000, 0.000000000000000000 ) ) ;
#2890=EDGE_LOOP ( 'NONE', ( #21573, #13156, #5085, #231 ) ) ;
#2897=VECTOR ( 'NONE', #19054, 1000.000000000000000 ) ;
#2903=CYLINDRICAL_SURFACE ( 'NONE', #16916, 5.249999999999942268 ) ;
#2908=ORIENTED_EDGE ( 'NONE', *, *, #18703, .F. ) ;
#2909=ORIENTED_EDGE ( 'NONE', *, *, #22120, .T. ) ;
#2924=VERTEX_POINT ( 'NONE', #11722 ) ;
#2939=DIRECTION ( 'NONE',  ( 0.000000000000000000, 0.000000000000000000, 1.000000000000000000 ) ) ;
#2958=B_SPLINE_CURVE_WITH_KNOTS ( 'NONE', 3,
 ( #8646, #68, #12662, #11072, #14561, #18391, #14803, #18177, #23715, #9122, #18277, #3546, #12546, #9004, #20205, #7170 ),
 .UNSPECIFIED., .F., .F.,
 ( 4, 2, 2, 2, 2, 2, 2, 4 ),
 ( 0.000000000000000000, 0.0009361184303669784889, 0.001404177645550537448, 0.001872236860734096623, 0.002340296075917655799, 0.002808355291101214540, 0.003276414506284773716, 0.003744473721468332891 ),
 .UNSPECIFIED. ) ;
#2959=ADVANCED_FACE ( 'NONE', ( #14964 ), #13662, .F. ) ;
#2965=CARTESIAN_POINT ( 'NONE',  ( -288.2000000000013529, -89.99999999999897682, 21.68333333333335844 ) ) ;
#2966=EDGE_CURVE ( 'NONE', #2924, #10594, #15323, .T. ) ;
#2969=DIRECTION ( 'NONE',  ( 0.000000000000000000, -1.000000000000000000, 0.000000000000000000 ) ) ;
#2970=CIRCLE ( 'NONE', #6066, 2.649999999999975486 ) ;
#2971=CARTESIAN_POINT ( 'NONE',  ( -283.1682701916307110, 271.9268706878666535, 145.6222583006965863 ) ) ;
#2975=CARTESIAN_POINT ( 'NONE',  ( -281.1815513148989112, 268.5095819834011763, -147.0873946496625422 ) ) ;
#2976=CARTESIAN_POINT ( 'NONE',  ( 280.6212670861564220, 269.5502846751310244, 146.3405375976306857 ) ) ;
#2983=CARTESIAN_POINT ( 'NONE',  ( 281.4928932188134354, -129.2000000000000455, -152.4000000000013131 ) ) ;
#2984=DIRECTION ( 'NONE',  ( 0.000000000000000000, 0.000000000000000000, 1.000000000000000000 ) ) ;
#2998=CARTESIAN_POINT ( 'NONE',  ( 281.4928932188134354, -127.0000000000000568, -147.2000000000013245 ) ) ;
#2999=VECTOR ( 'NONE', #7777, 1000.000000000000000 ) ;
#3001=ORIENTED_EDGE ( 'NONE', *, *, #10546, .T. ) ;
#3002=ADVANCED_FACE ( 'NONE', ( #16874 ), #20726, .F. ) ;
#3020=AXIS2_PLACEMENT_3D ( 'NONE', #4196, #8428, #20989 ) ;
#3024=FACE_BOUND ( 'NONE', #16999, .T. ) ;
#3027=FACE_OUTER_BOUND ( 'NONE', #20509, .T. ) ;
#3038=CARTESIAN_POINT ( 'NONE',  ( 281.4928932188134354, -129.2000000000000455, -177.2000000000013529 ) ) ;
#3039=DIRECTION ( 'NONE',  ( -0.000000000000000000, -0.000000000000000000, 1.000000000000000000 ) ) ;
#3043=AXIS2_PLACEMENT_3D ( 'NONE', #3870, #18482, #16682 ) ;
#3046=CARTESIAN_POINT ( 'NONE',  ( -281.0927021017107563, 269.6958543268121957, -145.4976310729377929 ) ) ;
#3048=ADVANCED_FACE ( 'NONE', ( #17950, #4912, #17585 ), #14237, .F. ) ;
#3062=AXIS2_PLACEMENT_3D ( 'NONE', #5301, #21831, #5534 ) ;
#3063=ORIENTED_EDGE ( 'NONE', *, *, #9786, .T. ) ;
#3064=DIRECTION ( 'NONE',  ( 1.000000000000000000, 3.495664435217746592E-15, -0.000000000000000000 ) ) ;
#3067=VECTOR ( 'NONE', #10793, 1000.000000000000000 ) ;
#3089=VECTOR ( 'NONE', #9119, 1000.000000000000000 ) ;
#3093=CARTESIAN_POINT ( 'NONE',  ( -287.4000000000014552, -129.2000000000000455, -146.4928932188134070 ) ) ;
#3095=DIRECTION ( 'NONE',  ( -0.000000000000000000, -0.000000000000000000, 1.000000000000000000 ) ) ;
#3102=FACE_OUTER_BOUND ( 'NONE', #22549, .T. ) ;
#3112=CARTESIAN_POINT ( 'NONE',  ( 281.1815513148990817, 268.5095819834012332, 147.0873946496626274 ) ) ;
#3118=CYLINDRICAL_SURFACE ( 'NONE', #11040, 2.199999999999979750 ) ;
#3136=DIRECTION ( 'NONE',  ( 0.000000000000000000, -0.000000000000000000, 1.000000000000000000 ) ) ;
#3138=CARTESIAN_POINT ( 'NONE',  ( 285.2000000000013529, -127.0000000000000568, 0.000000000000000000 ) ) ;
#3140=FACE_OUTER_BOUND ( 'NONE', #430, .T. ) ;
#3141=ORIENTED_EDGE ( 'NONE', *, *, #14682, .T. ) ;
#3143=DIRECTION ( 'NONE',  ( -1.000000000000000000, 3.495664435217746592E-15, -0.000000000000000000 ) ) ;
#3146=EDGE_LOOP ( 'NONE', ( #10561, #13581, #1185, #10583 ) ) ;
#3151=CARTESIAN_POINT ( 'NONE',  ( -280.0627656775836840, 269.9999999999999432, 145.1452901038202015 ) ) ;
#3192=CYLINDRICAL_SURFACE ( 'NONE', #18803, 5.249999999999973355 ) ;
#3221=AXIS2_PLACEMENT_3D ( 'NONE', #11449, #13391, #1992 ) ;
#3233=ORIENTED_EDGE ( 'NONE', *, *, #17686, .T. ) ;
#3237=EDGE_CURVE ( 'NONE', #15299, #12940, #9016, .T. ) ;
#3250=EDGE_CURVE ( 'NONE', #20963, #11281, #10779, .T. ) ;
#3262=ORIENTED_EDGE ( 'NONE', *, *, #22699, .F. ) ;
#3268=DIRECTION ( 'NONE',  ( 1.000000000000000000, 0.000000000000000000, 0.000000000000000000 ) ) ;
#3274=ORIENTED_EDGE ( 'NONE', *, *, #16709, .T. ) ;
#3280=ADVANCED_FACE ( 'NONE', ( #23213 ), #6921, .F. ) ;
#3286=ORIENTED_EDGE ( 'NONE', *, *, #6247, .T. ) ;
#3311=DIRECTION ( 'NONE',  ( 0.000000000000000000, -1.000000000000000000, 0.000000000000000000 ) ) ;
#3314=CARTESIAN_POINT ( 'NONE',  ( -285.2300000000000182, 268.4847249064869743, 146.3684637172358691 ) ) ;
#3318=ORIENTED_EDGE ( 'NONE', *, *, #12480, .F. ) ;
#3339=ORIENTED_EDGE ( 'NONE', *, *, #12855, .T. ) ;
#3345=LINE ( 'NONE', #11462, #16373 ) ;
#3355=VERTEX_POINT ( 'NONE', #21401 ) ;
#3356=ORIENTED_EDGE ( 'NONE', *, *, #12322, .F. ) ;
#3363=CYLINDRICAL_SURFACE ( 'NONE', #21096, 2.649999999999971934 ) ;
#3364=AXIS2_PLACEMENT_3D ( 'NONE', #9388, #12921, #5511 ) ;
#3368=CARTESIAN_POINT ( 'NONE',  ( -287.4000000000014552, -127.0000000000000568, -146.4928932188134070 ) ) ;
#3371=EDGE_LOOP ( 'NONE', ( #19340, #19857, #830, #21633 ) ) ;
#3379=DIRECTION ( 'NONE',  ( 0.000000000000000000, -4.183096374613631247E-18, 1.000000000000000000 ) ) ;
#3383=CYLINDRICAL_SURFACE ( 'NONE', #13473, 2.649999999999971934 ) ;
#3388=CYLINDRICAL_SURFACE ( 'NONE', #8399, 2.649999999999971934 ) ;
#3393=DIRECTION ( 'NONE',  ( 0.000000000000000000, -0.000000000000000000, 1.000000000000000000 ) ) ;
#3396=CIRCLE ( 'NONE', #18817, 2.199999999999979750 ) ;
#3406=ADVANCED_FACE ( 'NONE', ( #5141 ), #2842, .F. ) ;
#3409=AXIS2_PLACEMENT_3D ( 'NONE', #4191, #340, #11608 ) ;
#3417=CARTESIAN_POINT ( 'NONE',  ( -282.2000000000012960, -74.99999999999899103, 90.00000000000000000 ) ) ;
#3428=AXIS2_PLACEMENT_3D ( 'NONE', #9803, #845, #11760 ) ;
#3436=CARTESIAN_POINT ( 'NONE',  ( -281.3333820183296439, 269.5350371479512432, 145.6220388411722695 ) ) ;
#3438=VECTOR ( 'NONE', #13932, 1000.000000000000000 ) ;
#3441=CARTESIAN_POINT ( 'NONE',  ( 281.3683070494394087, 268.4816199723481986, -150.1663417894421571 ) ) ;
#3442=VECTOR ( 'NONE', #13251, 1000.000000000000000 ) ;
#3454=DIRECTION ( 'NONE',  ( -3.495664435217746987E-15, 1.000000000000000000, 0.000000000000000000 ) ) ;
#3458=CARTESIAN_POINT ( 'NONE',  ( 282.2000000000013529, -127.0000000000000568, -146.4928932188134070 ) ) ;
#3459=CARTESIAN_POINT ( 'NONE',  ( -281.4928932188135491, -132.2000000000000455, 152.4000000000014268 ) ) ;
#3460=FACE_OUTER_BOUND ( 'NONE', #12390, .T. ) ;
#3462=ORIENTED_EDGE ( 'NONE', *, *, #14840, .T. ) ;
#3469=ORIENTED_EDGE ( 'NONE', *, *, #22005, .T. ) ;
#3474=CARTESIAN_POINT ( 'NONE',  ( 280.8708543776410806, 269.1520027839447948, 146.7592670532760053 ) ) ;
#3493=ORIENTED_EDGE ( 'NONE', *, *, #2966, .F. ) ;
#3504=DIRECTION ( 'NONE',  ( -0.000000000000000000, -0.000000000000000000, -1.000000000000000000 ) ) ;
#3511=FACE_OUTER_BOUND ( 'NONE', #8305, .T. ) ;
#3515=EDGE_CURVE ( 'NONE', #10685, #3355, #11779, .T. ) ;
#3533=CARTESIAN_POINT ( 'NONE',  ( -34.75000000000005684, 100.0000000000000000, 150.2000000000009550 ) ) ;
#3534=EDGE_CURVE ( 'NONE', #19310, #15178, #14926, .T. ) ;
#3536=CARTESIAN_POINT ( 'NONE',  ( 281.4928932188133217, -127.0000000000000568, 152.4000000000014268 ) ) ;
#3546=CARTESIAN_POINT ( 'NONE',  ( 280.3113419039144105, 269.8873946496627809, -145.7095819834011650 ) ) ;
#3549=CARTESIAN_POINT ( 'NONE',  ( -281.3610889986683219, 272.8646579186752774, 145.2488155364689248 ) ) ;
#3554=VERTEX_POINT ( 'NONE', #11209 ) ;
#3556=CARTESIAN_POINT ( 'NONE',  ( -281.4928932188135491, -127.0000000000000568, 147.2000000000013813 ) ) ;
#3560=DIRECTION ( 'NONE',  ( -1.000000000000000000, 0.000000000000000000, 0.000000000000000000 ) ) ;
#3585=DIRECTION ( 'NONE',  ( -1.000000000000000000, 3.495664435217746987E-15, 0.000000000000000000 ) ) ;
#3595=VERTEX_POINT ( 'NONE', #18527 ) ;
#3596=CARTESIAN_POINT ( 'NONE',  ( 281.4928932188133786, 5.173457871231061435E-13, 150.2000000000009550 ) ) ;
#3598=DIRECTION ( 'NONE',  ( 0.000000000000000000, -3.495664435217746987E-15, 1.000000000000000000 ) ) ;
#3605=VECTOR ( 'NONE', #9548, 1000.000000000000000 ) ;
#3608=VERTEX_POINT ( 'NONE', #5611 ) ;
#3609=DIRECTION ( 'NONE',  ( 0.000000000000000000, -1.000000000000000000, -0.000000000000000000 ) ) ;
#3613=VERTEX_POINT ( 'NONE', #3908 ) ;
#3619=ORIENTED_EDGE ( 'NONE', *, *, #4415, .T. ) ;
#3622=CARTESIAN_POINT ( 'NONE',  ( 99.99999999999987210, -127.0000000000000568, 152.4000000000014268 ) ) ;
#3627=CYLINDRICAL_SURFACE ( 'NONE', #12248, 5.249999999999942268 ) ;
#3632=CARTESIAN_POINT ( 'NONE',  ( 312.2000000000013529, -129.2000000000000455, 146.4928932188134638 ) ) ;
#3646=DIRECTION ( 'NONE',  ( 0.000000000000000000, -1.000000000000000000, 0.000000000000000000 ) ) ;
#3647=LINE ( 'NONE', #7521, #3442 ) ;
#3655=EDGE_CURVE ( 'NONE', #22159, #6854, #18918, .T. ) ;
#3656=DIRECTION ( 'NONE',  ( 0.000000000000000000, -1.000000000000000000, 0.000000000000000000 ) ) ;
#3659=AXIS2_PLACEMENT_3D ( 'NONE', #12726, #21737, #5197 ) ;
#3660=DIRECTION ( 'NONE',  ( -0.000000000000000000, 1.000000000000000000, -0.000000000000000000 ) ) ;
#3667=DIRECTION ( 'NONE',  ( 1.000000000000000000, -0.000000000000000000, -0.000000000000000000 ) ) ;
#3671=ADVANCED_FACE ( 'NONE', ( #15291 ), #8161, .F. ) ;
#3683=CARTESIAN_POINT ( 'NONE',  ( -285.2000000000013529, -89.99999999999896261, -37.68333333333335844 ) ) ;
#3687=CYLINDRICAL_SURFACE ( 'NONE', #11234, 5.199999999999982414 ) ;
#3691=FACE_OUTER_BOUND ( 'NONE', #20690, .T. ) ;
#3709=AXIS2_PLACEMENT_3D ( 'NONE', #16694, #20293, #22468 ) ;
#3734=VECTOR ( 'NONE', #2394, 1000.000000000000000 ) ;
#3738=PLANE ( 'NONE',  #11551 ) ;
#3739=VERTEX_POINT ( 'NONE', #6929 ) ;
#3740=DIRECTION ( 'NONE',  ( 1.000000000000000000, -3.491481338843133355E-15, 0.000000000000000000 ) ) ;
#3741=VECTOR ( 'NONE', #7148, 1000.000000000000000 ) ;
#3745=ORIENTED_EDGE ( 'NONE', *, *, #1516, .T. ) ;
#3748=CARTESIAN_POINT ( 'NONE',  ( 280.1244294735509470, 273.0000000000000000, -145.6807971656550933 ) ) ;
#3752=AXIS2_PLACEMENT_3D ( 'NONE', #10984, #18303, #9147 ) ;
#3754=ORIENTED_EDGE ( 'NONE', *, *, #10151, .T. ) ;
#3760=VECTOR ( 'NONE', #625, 1000.000000000000000 ) ;
#3762=EDGE_LOOP ( 'NONE', ( #17911, #2104, #2310, #10511 ) ) ;
#3763=CARTESIAN_POINT ( 'NONE',  ( -282.2000000000007276, 75.00000000000100897, -90.00000000000000000 ) ) ;
#3769=DIRECTION ( 'NONE',  ( 1.000000000000000000, 0.000000000000000000, 0.000000000000000000 ) ) ;
#3783=CARTESIAN_POINT ( 'NONE',  ( -280.3431883596742864, 273.0000000000000000, -145.0627246250092810 ) ) ;
#3787=AXIS2_PLACEMENT_3D ( 'NONE', #18219, #9303, #18563 ) ;
#3794=ORIENTED_EDGE ( 'NONE', *, *, #185, .F. ) ;
#3798=PLANE ( 'NONE',  #16191 ) ;
#3807=CARTESIAN_POINT ( 'NONE',  ( 279.9999999999999432, 272.9999999999999432, 145.0000000000000284 ) ) ;
#3808=EDGE_CURVE ( 'NONE', #6854, #15324, #5003, .T. ) ;
#3809=EDGE_CURVE ( 'NONE', #9091, #4872, #2677, .T. ) ;
#3812=CARTESIAN_POINT ( 'NONE',  ( 285.2000000000013529, -127.0000000000000568, 146.4928932188134638 ) ) ;
#3820=CARTESIAN_POINT ( 'NONE',  ( 282.1999999999999318, 267.7999999999999545, -146.4928932188133786 ) ) ;
#3825=DIRECTION ( 'NONE',  ( 1.000000000000000000, -0.000000000000000000, -9.860133695827843917E-17 ) ) ;
#3827=PLANE ( 'NONE',  #16196 ) ;
#3830=DIRECTION ( 'NONE',  ( 0.000000000000000000, -1.000000000000000000, -3.172065784643303781E-15 ) ) ;
#3837=VECTOR ( 'NONE', #17919, 1000.000000000000000 ) ;
#3846=DIRECTION ( 'NONE',  ( 0.000000000000000000, 1.000000000000000000, -3.495664435217746987E-15 ) ) ;
#3851=CARTESIAN_POINT ( 'NONE',  ( -281.4928932188134354, 35.00000000000022737, 147.2000000000008413 ) ) ;
#3862=ORIENTED_EDGE ( 'NONE', *, *, #15221, .F. ) ;
#3864=ORIENTED_EDGE ( 'NONE', *, *, #11275, .T. ) ;
#3866=CARTESIAN_POINT ( 'NONE',  ( -45.00000000000000000, 272.9999999999999432, 0.000000000000000000 ) ) ;
#3870=CARTESIAN_POINT ( 'NONE',  ( 0.000000000000000000, -129.2000000000000455, 7.690461757479017101E-15 ) ) ;
#3873=FACE_OUTER_BOUND ( 'NONE', #19383, .T. ) ;
#3874=CARTESIAN_POINT ( 'NONE',  ( 281.4928932188134354, -132.2000000000000455, -7.703011046602857601E-15 ) ) ;
#3899=CARTESIAN_POINT ( 'NONE',  ( -280.4976310729378497, 272.3699028110927429, -147.6339272673398000 ) ) ;
#3901=ORIENTED_EDGE ( 'NONE', *, *, #9449, .T. ) ;
#3905=CARTESIAN_POINT ( 'NONE',  ( 281.1079617568158824, 269.7223300543793698, 145.4976310729378497 ) ) ;
#3908=CARTESIAN_POINT ( 'NONE',  ( -282.2000000000013529, -89.99999999999896261, -37.68333333333335844 ) ) ;
#3926=DIRECTION ( 'NONE',  ( -0.000000000000000000, -0.000000000000000000, 1.000000000000000000 ) ) ;
#3930=DIRECTION ( 'NONE',  ( 0.000000000000000000, -1.000000000000000000, 0.000000000000000000 ) ) ;
#3937=DIRECTION ( 'NONE',  ( 0.000000000000000000, 1.000000000000000000, 4.183096374613631247E-18 ) ) ;
#3942=DIRECTION ( 'NONE',  ( -0.000000000000000000, 1.000000000000000000, 0.000000000000000000 ) ) ;
#3944=ORIENTED_EDGE ( 'NONE', *, *, #20619, .F. ) ;
#3949=ORIENTED_EDGE ( 'NONE', *, *, #8706, .F. ) ;
#3952=PLANE ( 'NONE',  #22944 ) ;
#3957=CYLINDRICAL_SURFACE ( 'NONE', #9933, 2.649999999999971934 ) ;
#3959=CARTESIAN_POINT ( 'NONE',  ( -288.2000000000006708, 90.00000000000102318, -35.00000000000001421 ) ) ;
#3965=VERTEX_POINT ( 'NONE', #22112 ) ;
#3967=VECTOR ( 'NONE', #23784, 1000.000000000000000 ) ;
#3968=EDGE_CURVE ( 'NONE', #17073, #15945, #7270, .T. ) ;
#3971=DIRECTION ( 'NONE',  ( -1.000000000000000000, 0.000000000000000000, 0.000000000000000000 ) ) ;
#3972=DIRECTION ( 'NONE',  ( 0.000000000000000000, 0.000000000000000000, -1.000000000000000000 ) ) ;
#3980=FILL_AREA_STYLE_COLOUR ( '', #16226 ) ;
#3998=EDGE_LOOP ( 'NONE', ( #17400, #15518 ) ) ;
#4007=CARTESIAN_POINT ( 'NONE',  ( -280.1244266425809428, 269.9697000000000457, -145.2840560642351875 ) ) ;
#4013=DIRECTION ( 'NONE',  ( -1.000000000000000000, 0.000000000000000000, 0.000000000000000000 ) ) ;
#4015=CARTESIAN_POINT ( 'NONE',  ( 282.1696999999999775, 268.0840560642351988, 146.3684665762324926 ) ) ;
#4016=CARTESIAN_POINT ( 'NONE',  ( -285.2000000000000455, 267.7999999999999545, -146.4928932188134354 ) ) ;
#4019=CARTESIAN_POINT ( 'NONE',  ( -281.4928932188134354, -127.0000000000000568, -152.4000000000012847 ) ) ;
#4025=VERTEX_POINT ( 'NONE', #2182 ) ;
#4032=CARTESIAN_POINT ( 'NONE',  ( 279.9999999999999432, 269.9999999999999432, 145.0000000000000284 ) ) ;
#4045=VERTEX_POINT ( 'NONE', #11299 ) ;
#4046=VECTOR ( 'NONE', #20463, 1000.000000000000000 ) ;
#4052=AXIS2_PLACEMENT_3D ( 'NONE', #12201, #3095, #14117 ) ;
#4066=ADVANCED_FACE ( 'NONE', ( #7627 ), #19087, .F. ) ;
#4097=LINE ( 'NONE', #17046, #746 ) ;
#4098=ORIENTED_EDGE ( 'NONE', *, *, #14078, .T. ) ;
#4100=FACE_BOUND ( 'NONE', #5634, .T. ) ;
#4104=LINE ( 'NONE', #6045, #2309 ) ;
#4106=CARTESIAN_POINT ( 'NONE',  ( 281.3684637172358975, 268.4847249064869175, -150.2299999999999329 ) ) ;
#4108=ORIENTED_EDGE ( 'NONE', *, *, #5599, .F. ) ;
#4120=FACE_OUTER_BOUND ( 'NONE', #14104, .T. ) ;
#4123=DIRECTION ( 'NONE',  ( -0.000000000000000000, 1.000000000000000000, -0.000000000000000000 ) ) ;
#4129=CARTESIAN_POINT ( 'NONE',  ( -280.8708543776411943, 269.1520027839447948, -146.7592670532759769 ) ) ;
#4138=CARTESIAN_POINT ( 'NONE',  ( 281.9223300543793584, 268.9079617568158938, 145.9952621458756710 ) ) ;
#4141=AXIS2_PLACEMENT_3D ( 'NONE', #10693, #5112, #16452 ) ;
#4143=AXIS2_PLACEMENT_3D ( 'NONE', #17218, #4161, #22867 ) ;
#4147=FACE_OUTER_BOUND ( 'NONE', #17080, .T. ) ;
#4151=EDGE_LOOP ( 'NONE', ( #2618, #11876, #12754, #15577 ) ) ;
#4154=LINE ( 'NONE', #22394, #1378 ) ;
#4161=DIRECTION ( 'NONE',  ( -0.000000000000000000, 1.000000000000000000, -0.000000000000000000 ) ) ;
#4167=LINE ( 'NONE', #559, #8864 ) ;
#4178=DIRECTION ( 'NONE',  ( 0.000000000000000000, 0.000000000000000000, -1.000000000000000000 ) ) ;
#4179=CIRCLE ( 'NONE', #6120, 2.649999999999971934 ) ;
#4184=EDGE_CURVE ( 'NONE', #10594, #14150, #2506, .T. ) ;
#4186=CIRCLE ( 'NONE', #5345, 2.649999999999971934 ) ;
#4190=CYLINDRICAL_SURFACE ( 'NONE', #5602, 2.199999999999979750 ) ;
#4191=CARTESIAN_POINT ( 'NONE',  ( -288.2000000000008981, 30.00000000000101963, -105.0000000000000142 ) ) ;
#4195=FACE_BOUND ( 'NONE', #9545, .T. ) ;
#4196=CARTESIAN_POINT ( 'NONE',  ( 99.99999999999987210, -127.0000000000000568, 152.4000000000014268 ) ) ;
#4205=CARTESIAN_POINT ( 'NONE',  ( 282.2000000000013529, -127.0000000000000568, -146.4928932188134070 ) ) ;
#4207=AXIS2_PLACEMENT_3D ( 'NONE', #4231, #500, #13695 ) ;
#4218=DIRECTION ( 'NONE',  ( -0.000000000000000000, 1.000000000000000000, 3.495664435217746987E-15 ) ) ;
#4220=ORIENTED_EDGE ( 'NONE', *, *, #12562, .F. ) ;
#4222=CARTESIAN_POINT ( 'NONE',  ( -100.0000000000000000, 35.00000000000009948, 147.2000000000008413 ) ) ;
#4228=CARTESIAN_POINT ( 'NONE',  ( 283.4379565153277554, 271.7159870726002850, 145.6846668451111952 ) ) ;
#4231=CARTESIAN_POINT ( 'NONE',  ( -40.00000000000000000, 100.0000000000000000, 147.2000000000005855 ) ) ;
#4233=DIRECTION ( 'NONE',  ( 1.000000000000000000, -0.000000000000000000, -0.000000000000000000 ) ) ;
#4239=DIRECTION ( 'NONE',  ( -0.000000000000000000, 7.709882115452476934E-17, -1.000000000000000000 ) ) ;
#4240=CARTESIAN_POINT ( 'NONE',  ( 280.4976310729377929, 269.7223300543794267, -146.1079617568159392 ) ) ;
#4250=CARTESIAN_POINT ( 'NONE',  ( 285.1999999999999318, 267.7999999999999545, -146.4928932188133786 ) ) ;
#4253=CARTESIAN_POINT ( 'NONE',  ( -280.6220388411723548, 269.5592670532759030, 146.3520027839448119 ) ) ;
#4265=VECTOR ( 'NONE', #3039, 1000.000000000000000 ) ;
#4269=CARTESIAN_POINT ( 'NONE',  ( -282.2000000000000455, 267.7999999999999545, 146.4928932188134354 ) ) ;
#4272=ORIENTED_EDGE ( 'NONE', *, *, #2812, .F. ) ;
#4273=ORIENTED_EDGE ( 'NONE', *, *, #21790, .T. ) ;
#4277=FACE_OUTER_BOUND ( 'NONE', #12268, .T. ) ;
#4281=CARTESIAN_POINT ( 'NONE',  ( 281.4928932188134354, -132.2000000000000455, -177.2000000000013529 ) ) ;
#4284=ORIENTED_EDGE ( 'NONE', *, *, #9177, .T. ) ;
#4293=ORIENTED_EDGE ( 'NONE', *, *, #15282, .F. ) ;
#4309=VERTEX_POINT ( 'NONE', #12965 ) ;
#4315=FACE_OUTER_BOUND ( 'NONE', #3762, .T. ) ;
#4318=CARTESIAN_POINT ( 'NONE',  ( 281.2434055557876036, 269.1518577254344677, 150.0327955282141374 ) ) ;
#4322=ORIENTED_EDGE ( 'NONE', *, *, #17266, .T. ) ;
#4323=CARTESIAN_POINT ( 'NONE',  ( 279.9999999999999432, 269.9696999999999889, -144.9999999999999716 ) ) ;
#4340=DIRECTION ( 'NONE',  ( -1.000000000000000000, -0.000000000000000000, -0.000000000000000000 ) ) ;
#4346=ORIENTED_EDGE ( 'NONE', *, *, #5933, .T. ) ;
#4350=CARTESIAN_POINT ( 'NONE',  ( 285.2000000000013529, -132.2000000000000455, 146.4928932188134638 ) ) ;
#4351=PLANE ( 'NONE',  #3428 ) ;
#4352=ORIENTED_EDGE ( 'NONE', *, *, #3237, .F. ) ;
#4355=( NAMED_UNIT ( * ) PLANE_ANGLE_UNIT ( ) SI_UNIT ( $, .RADIAN. ) );
#4356=VECTOR ( 'NONE', #13938, 1000.000000000000000 ) ;
#4368=CARTESIAN_POINT ( 'NONE',  ( -280.2488155364689533, 269.9427398886703031, 145.5758453455904373 ) ) ;
#4371=VECTOR ( 'NONE', #87, 1000.000000000000000 ) ;
#4377=CYLINDRICAL_SURFACE ( 'NONE', #19990, 2.649999999999971934 ) ;
#4388=CARTESIAN_POINT ( 'NONE',  ( 280.2840560642353012, 269.9696999999999889, 145.1244266425810849 ) ) ;
#4390=ORIENTED_EDGE ( 'NONE', *, *, #9505, .F. ) ;
#4396=VECTOR ( 'NONE', #12454, 1000.000000000000000 ) ;
#4399=PLANE ( 'NONE',  #14295 ) ;
#4415=EDGE_CURVE ( 'NONE', #10471, #2262, #20513, .T. ) ;
#4417=EDGE_CURVE ( 'NONE', #13591, #18466, #22448, .T. ) ;
#4424=CARTESIAN_POINT ( 'NONE',  ( 312.2000000000013529, -129.2000000000000455, 146.4928932188134638 ) ) ;
#4436=CARTESIAN_POINT ( 'NONE',  ( -100.0000000000000284, 5.837466857250891336E-13, 150.2000000000009550 ) ) ;
#4439=ORIENTED_EDGE ( 'NONE', *, *, #22344, .T. ) ;
#4440=DIRECTION ( 'NONE',  ( 4.183096374613631247E-18, 1.000000000000000000, -0.000000000000000000 ) ) ;
#4443=DIRECTION ( 'NONE',  ( 0.000000000000000000, 0.000000000000000000, -1.000000000000000000 ) ) ;
#4445=DIRECTION ( 'NONE',  ( -1.000000000000000000, 0.000000000000000000, 0.000000000000000000 ) ) ;
#4446=CIRCLE ( 'NONE', #5608, 5.249999999999949374 ) ;
#4454=VECTOR ( 'NONE', #2143, 1000.000000000000000 ) ;
#4461=FACE_OUTER_BOUND ( 'NONE', #22723, .T. ) ;
#4463=ORIENTED_EDGE ( 'NONE', *, *, #14055, .F. ) ;
#4470=ORIENTED_EDGE ( 'NONE', *, *, #23530, .T. ) ;
#4475=CIRCLE ( 'NONE', #19487, 2.199999999999979750 ) ;
#4476=FACE_OUTER_BOUND ( 'NONE', #23759, .T. ) ;
#4491=CARTESIAN_POINT ( 'NONE',  ( -281.3684665479256637, 268.0880230824753312, 147.1999999999999886 ) ) ;
#4508=CYLINDRICAL_SURFACE ( 'NONE', #23158, 5.249999999999973355 ) ;
#4518=DIRECTION ( 'NONE',  ( 0.000000000000000000, -3.495664435217746987E-15, 1.000000000000000000 ) ) ;
#4530=AXIS2_PLACEMENT_3D ( 'NONE', #16744, #1755, #12575 ) ;
#4570=AXIS2_PLACEMENT_3D ( 'NONE', #8965, #7134, #1342 ) ;
#4573=CARTESIAN_POINT ( 'NONE',  ( 280.9952621458755289, 270.4339272673396977, 149.5699028110927884 ) ) ;
#4576=ORIENTED_EDGE ( 'NONE', *, *, #20520, .T. ) ;
#4581=DIRECTION ( 'NONE',  ( 0.000000000000000000, -0.000000000000000000, 1.000000000000000000 ) ) ;
#4585=DIRECTION ( 'NONE',  ( -0.000000000000000000, -0.000000000000000000, 1.000000000000000000 ) ) ;
#4587=VECTOR ( 'NONE', #5751, 1000.000000000000000 ) ;
#4591=DIRECTION ( 'NONE',  ( -0.000000000000000000, 0.000000000000000000, -1.000000000000000000 ) ) ;
#4595=VERTEX_POINT ( 'NONE', #23171 ) ;
#4596=EDGE_CURVE ( 'NONE', #8654, #13423, #4446, .T. ) ;
#4611=CIRCLE ( 'NONE', #10812, 2.649999999999971934 ) ;
#4615=CARTESIAN_POINT ( 'NONE',  ( -280.8708543776413080, 271.0140793454687582, 149.1822575857424624 ) ) ;
#4622=ORIENTED_EDGE ( 'NONE', *, *, #7945, .F. ) ;
#4628=CIRCLE ( 'NONE', #5409, 5.199999999999982414 ) ;
#4630=VECTOR ( 'NONE', #14586, 1000.000000000000000 ) ;
#4635=EDGE_CURVE ( 'NONE', #23122, #5697, #22266, .T. ) ;
#4642=CARTESIAN_POINT ( 'NONE',  ( -284.5436892194422285, 270.4188186979286002, -145.9952621458756141 ) ) ;
#4643=VERTEX_POINT ( 'NONE', #16182 ) ;
#4651=LINE ( 'NONE', #9853, #5144 ) ;
#4654=CARTESIAN_POINT ( 'NONE',  ( 281.4928932188134354, 5.173457871231059415E-13, -150.2000000000008981 ) ) ;
#4655=ORIENTED_EDGE ( 'NONE', *, *, #21263, .T. ) ;
#4662=CYLINDRICAL_SURFACE ( 'NONE', #11988, 2.199999999999979750 ) ;
#4680=DIRECTION ( 'NONE',  ( 0.000000000000000000, -0.000000000000000000, 1.000000000000000000 ) ) ;
#4687=DIRECTION ( 'NONE',  ( 0.000000000000000000, 0.000000000000000000, 1.000000000000000000 ) ) ;
#4694=ORIENTED_EDGE ( 'NONE', *, *, #11717, .T. ) ;
#4696=EDGE_CURVE ( 'NONE', #2692, #17768, #6869, .T. ) ;
#4697=ORIENTED_EDGE ( 'NONE', *, *, #577, .T. ) ;
#4710=DIRECTION ( 'NONE',  ( -1.000000000000000000, -0.000000000000000000, -0.000000000000000000 ) ) ;
#4727=ORIENTED_EDGE ( 'NONE', *, *, #5550, .F. ) ;
#4732=DIRECTION ( 'NONE',  ( 0.000000000000000000, 1.000000000000000000, -5.286776307738891306E-15 ) ) ;
#4745=CARTESIAN_POINT ( 'NONE',  ( -280.2880230824754335, 269.9999999999999432, -145.1244266708878570 ) ) ;
#4755=LINE ( 'NONE', #7374, #3967 ) ;
#4757=LINE ( 'NONE', #13742, #8881 ) ;
#4766=PRODUCT ( 'head cover', 'head cover', '', ( #5785 ) ) ;
#4769=CARTESIAN_POINT ( 'NONE',  ( 280.1452901038202299, 270.0000000000000000, 145.0627656775837124 ) ) ;
#4777=ORIENTED_EDGE ( 'NONE', *, *, #7211, .F. ) ;
#4780=DIRECTION ( 'NONE',  ( -1.000000000000000000, -0.000000000000000000, -0.000000000000000000 ) ) ;
#4787=ORIENTED_EDGE ( 'NONE', *, *, #2304, .T. ) ;
#4792=ORIENTED_EDGE ( 'NONE', *, *, #18293, .F. ) ;
#4794=PLANE ( 'NONE',  #22645 ) ;
#4795=EDGE_CURVE ( 'NONE', #22159, #12385, #17089, .T. ) ;
#4820=ORIENTED_EDGE ( 'NONE', *, *, #11656, .T. ) ;
#4827=EDGE_CURVE ( 'NONE', #12111, #14699, #19000, .T. ) ;
#4828=CARTESIAN_POINT ( 'NONE',  ( 45.00000000000000000, 272.9999999999999432, 5.249999999999991118 ) ) ;
#4852=FACE_BOUND ( 'NONE', #10861, .T. ) ;
#4865=DIRECTION ( 'NONE',  ( -0.000000000000000000, 0.000000000000000000, -1.000000000000000000 ) ) ;
#4870=CARTESIAN_POINT ( 'NONE',  ( -283.1956429438696432, 271.9582675804705332, -145.6220388411722411 ) ) ;
#4872=VERTEX_POINT ( 'NONE', #20834 ) ;
#4878=CARTESIAN_POINT ( 'NONE',  ( -40.00000000000000000, 100.0000000000000000, 150.2000000000009550 ) ) ;
#4881=CARTESIAN_POINT ( 'NONE',  ( 45.00000000000000000, 272.9999999999999432, 0.000000000000000000 ) ) ;
#4883=LINE ( 'NONE', #18045, #23251 ) ;
#4888=CYLINDRICAL_SURFACE ( 'NONE', #10412, 2.649999999999971934 ) ;
#4889=EDGE_CURVE ( 'NONE', #14699, #6854, #19245, .T. ) ;
#4891=EDGE_CURVE ( 'NONE', #5697, #8918, #11432, .T. ) ;
#4912=FACE_BOUND ( 'NONE', #15438, .T. ) ;
#4922=CARTESIAN_POINT ( 'NONE',  ( 281.4928932188133786, -132.2000000000000455, 177.2000000000014097 ) ) ;
#4926=CARTESIAN_POINT ( 'NONE',  ( -281.4928932188134354, 267.8000000000000114, -147.1999999999999318 ) ) ;
#4932=EDGE_CURVE ( 'NONE', #22646, #5795, #9894, .T. ) ;
#4939=DIRECTION ( 'NONE',  ( -0.000000000000000000, -1.000000000000000000, -0.000000000000000000 ) ) ;
#4946=ORIENTED_EDGE ( 'NONE', *, *, #15372, .F. ) ;
#4950=CARTESIAN_POINT ( 'NONE',  ( -281.4928932188134354, 267.8000000000000114, -150.1999999999999318 ) ) ;
#4955=CARTESIAN_POINT ( 'NONE',  ( -288.2000000000011255, -29.99999999999898037, -105.0000000000000000 ) ) ;
#4960=EDGE_LOOP ( 'NONE', ( #11267, #9945, #18260, #19474 ) ) ;
#4963=ORIENTED_EDGE ( 'NONE', *, *, #7945, .T. ) ;
#4967=CIRCLE ( 'NONE', #3787, 5.249999999999949374 ) ;
#4979=CARTESIAN_POINT ( 'NONE',  ( -35.00000000000000711, 4.286263797015737285E-15, -177.2000000000013529 ) ) ;
#4993=VECTOR ( 'NONE', #9692, 1000.000000000000000 ) ;
#5003=LINE ( 'NONE', #6443, #21197 ) ;
#5006=VERTEX_POINT ( 'NONE', #10701 ) ;
#5022=CARTESIAN_POINT ( 'NONE',  ( -285.2000000000008981, 30.00000000000101963, -102.3500000000000369 ) ) ;
#5029=ORIENTED_EDGE ( 'NONE', *, *, #11277, .T. ) ;
#5038=FACE_OUTER_BOUND ( 'NONE', #6189, .T. ) ;
#5041=EDGE_LOOP ( 'NONE', ( #2123, #3141, #18929, #11376 ) ) ;
#5043=ADVANCED_FACE ( 'NONE', ( #23591 ), #16117, .F. ) ;
#5047=LINE ( 'NONE', #3556, #4396 ) ;
#5051=CARTESIAN_POINT ( 'NONE',  ( 285.2000000000013529, -127.0000000000000568, -146.4928932188134070 ) ) ;
#5053=CARTESIAN_POINT ( 'NONE',  ( -35.00000000000000711, 4.286263797015349166E-15, -147.2000000000008981 ) ) ;
#5061=CARTESIAN_POINT ( 'NONE',  ( 281.3673129565597151, 268.0906609804447385, 147.1854425596106921 ) ) ;
#5066=CARTESIAN_POINT ( 'NONE',  ( 281.4928932188133217, 267.7999999999999545, 150.2299999999999898 ) ) ;
#5067=CARTESIAN_POINT ( 'NONE',  ( -45.00000000000000000, 269.9999999999999432, 0.000000000000000000 ) ) ;
#5071=DIRECTION ( 'NONE',  ( -0.000000000000000000, -0.000000000000000000, 1.000000000000000000 ) ) ;
#5072=EDGE_LOOP ( 'NONE', ( #21356, #3944, #6775, #20068 ) ) ;
#5077=CARTESIAN_POINT ( 'NONE',  ( -281.3681929792554115, 268.4822561791010003, -150.1663407402828909 ) ) ;
#5085=ORIENTED_EDGE ( 'NONE', *, *, #6210, .T. ) ;
#5087=LINE ( 'NONE', #21846, #20686 ) ;
#5088=EDGE_LOOP ( 'NONE', ( #1020, #15111, #16638, #3063, #3619, #20428, #19414, #20248 ) ) ;
#5090=B_SPLINE_CURVE_WITH_KNOTS ( 'NONE', 3,
 ( #823, #6621, #19289, #2853, #14250, #2753, #12462, #17844, #2971, #23390, #10255, #8558, #8429, #15689, #22901, #10509, #17594, #1049, #19762, #21343 ),
 .UNSPECIFIED., .F., .F.,
 ( 4, 2, 2, 2, 2, 2, 2, 2, 2, 4 ),
 ( 0.000000000000000000, 0.001035985217005883649, 0.002071970434011767299, 0.003107955651017651165, 0.003625948259520570330, 0.004143940868023489495, 0.005179926085029110984, 0.006215911302034731606, 0.007251896519040352228, 0.008287881736045972850 ),
 .UNSPECIFIED. ) ;
#5099=CARTESIAN_POINT ( 'NONE',  ( 99.99999999999987210, -129.2000000000000455, 152.4000000000014268 ) ) ;
#5100=ORIENTED_EDGE ( 'NONE', *, *, #23412, .F. ) ;
#5101=PLANE ( 'NONE',  #678 ) ;
#5104=EDGE_LOOP ( 'NONE', ( #4220, #18245, #19362, #17110 ) ) ;
#5112=DIRECTION ( 'NONE',  ( 0.000000000000000000, 0.000000000000000000, -1.000000000000000000 ) ) ;
#5119=ORIENTED_EDGE ( 'NONE', *, *, #8437, .F. ) ;
#5122=EDGE_LOOP ( 'NONE', ( #14317, #14513, #3462, #9489 ) ) ;
#5123=CARTESIAN_POINT ( 'NONE',  ( -280.8706349181170481, 270.9682701916305518, 149.1268706878666706 ) ) ;
#5129=EDGE_CURVE ( 'NONE', #3613, #23122, #19882, .T. ) ;
#5135=VECTOR ( 'NONE', #17355, 1000.000000000000000 ) ;
#5136=EDGE_LOOP ( 'NONE', ( #19706, #11947, #11406, #8098 ) ) ;
#5137=DIRECTION ( 'NONE',  ( 1.000000000000000000, -3.495664435217746987E-15, -0.000000000000000000 ) ) ;
#5139=CARTESIAN_POINT ( 'NONE',  ( -282.1697000000000912, 267.7999999999999545, 146.4928932188134354 ) ) ;
#5140=CARTESIAN_POINT ( 'NONE',  ( -100.0000000000000000, 35.00000000000009948, -113.4834095219707848 ) ) ;
#5141=FACE_OUTER_BOUND ( 'NONE', #13713, .T. ) ;
#5144=VECTOR ( 'NONE', #15534, 1000.000000000000000 ) ;
#5145=ORIENTED_EDGE ( 'NONE', *, *, #18703, .T. ) ;
#5146=LINE ( 'NONE', #23615, #12616 ) ;
#5154=LINE ( 'NONE', #3458, #12910 ) ;
#5160=VERTEX_POINT ( 'NONE', #15024 ) ;
#5161=CYLINDRICAL_SURFACE ( 'NONE', #3364, 2.649999999999971934 ) ;
#5162=DIRECTION ( 'NONE',  ( 1.000000000000000000, 0.000000000000000000, 0.000000000000000000 ) ) ;
#5177=ORIENTED_EDGE ( 'NONE', *, *, #20562, .F. ) ;
#5188=DIRECTION ( 'NONE',  ( 0.000000000000000000, -1.000000000000000000, 0.000000000000000000 ) ) ;
#5191=EDGE_LOOP ( 'NONE', ( #22391, #352, #7597, #5517 ) ) ;
#5197=DIRECTION ( 'NONE',  ( -1.000000000000000000, 0.000000000000000000, -0.000000000000000000 ) ) ;
#5200=ADVANCED_FACE ( 'NONE', ( #862, #17182, #4120 ), #20666, .F. ) ;
#5210=CARTESIAN_POINT ( 'NONE',  ( -280.9954397628185916, 268.9021437883071712, 146.9094021484633856 ) ) ;
#5215=DIRECTION ( 'NONE',  ( 0.000000000000000000, 1.000000000000000000, -4.183096374613631247E-18 ) ) ;
#5221=EDGE_LOOP ( 'NONE', ( #16159, #9471, #6726, #17758 ) ) ;
#5224=DIRECTION ( 'NONE',  ( 0.000000000000000000, 0.000000000000000000, 1.000000000000000000 ) ) ;
#5258=CIRCLE ( 'NONE', #10281, 2.649999999999978595 ) ;
#5269=CARTESIAN_POINT ( 'NONE',  ( -288.2000000000013529, -89.99999999999897682, 24.33333333333333215 ) ) ;
#5282=DIRECTION ( 'NONE',  ( 0.000000000000000000, 0.000000000000000000, -1.000000000000000000 ) ) ;
#5284=EDGE_LOOP ( 'NONE', ( #10922, #18845, #2299, #18557 ) ) ;
#5288=EDGE_LOOP ( 'NONE', ( #18687, #1653, #22937, #6586 ) ) ;
#5294=CARTESIAN_POINT ( 'NONE',  ( 281.4928932188134354, -132.2000000000000455, -152.4000000000012847 ) ) ;
#5301=CARTESIAN_POINT ( 'NONE',  ( 0.000000000000000000, 0.000000000000000000, -177.2000000000013529 ) ) ;
#5305=EDGE_LOOP ( 'NONE', ( #17054, #16245 ) ) ;
#5310=CIRCLE ( 'NONE', #4141, 2.199999999999979750 ) ;
#5320=CIRCLE ( 'NONE', #20333, 5.249999999999962697 ) ;
#5323=LINE ( 'NONE', #14520, #18495 ) ;
#5324=AXIS2_PLACEMENT_3D ( 'NONE', #20521, #3972, #18700 ) ;
#5335=EDGE_CURVE ( 'NONE', #10559, #17412, #15731, .T. ) ;
#5337=VERTEX_POINT ( 'NONE', #10300 ) ;
#5345=AXIS2_PLACEMENT_3D ( 'NONE', #10944, #21887, #5358 ) ;
#5356=CARTESIAN_POINT ( 'NONE',  ( -280.2494876630257750, 272.8327955282141488, 146.3518577254344279 ) ) ;
#5358=DIRECTION ( 'NONE',  ( 0.000000000000000000, -1.000000000000000000, 0.000000000000000000 ) ) ;
#5366=CARTESIAN_POINT ( 'NONE',  ( 279.9999999999999432, 269.9999999999999432, 145.0000000000000284 ) ) ;
#5375=ORIENTED_EDGE ( 'NONE', *, *, #2311, .F. ) ;
#5378=CARTESIAN_POINT ( 'NONE',  ( -281.8958543268122980, 268.8927021017106540, 145.9952621458756425 ) ) ;
#5386=VERTEX_POINT ( 'NONE', #2791 ) ;
#5388=VECTOR ( 'NONE', #9750, 1000.000000000000000 ) ;
#5389=CARTESIAN_POINT ( 'NONE',  ( -312.2000000000014666, -132.2000000000000455, -146.4928932188134070 ) ) ;
#5390=VERTEX_POINT ( 'NONE', #15619 ) ;
#5392=CARTESIAN_POINT ( 'NONE',  ( 285.2000000000008981, 9.892604858775018348E-13, -146.4928932188134070 ) ) ;
#5396=DIRECTION ( 'NONE',  ( -1.000000000000000000, -0.000000000000000000, -0.000000000000000000 ) ) ;
#5397=DIRECTION ( 'NONE',  ( -1.000000000000000000, -0.000000000000000000, -0.000000000000000000 ) ) ;
#5398=CARTESIAN_POINT ( 'NONE',  ( -281.4928932188135491, -129.2000000000000455, 152.4000000000014268 ) ) ;
#5409=AXIS2_PLACEMENT_3D ( 'NONE', #11677, #4013, #18984 ) ;
#5415=ORIENTED_EDGE ( 'NONE', *, *, #19779, .F. ) ;
#5416=CARTESIAN_POINT ( 'NONE',  ( 281.4928932188133217, 267.7999999999999545, 147.1999999999999886 ) ) ;
#5425=ORIENTED_EDGE ( 'NONE', *, *, #5592, .T. ) ;
#5426=EDGE_LOOP ( 'NONE', ( #10632, #3949 ) ) ;
#5448=CARTESIAN_POINT ( 'NONE',  ( 0.000000000000000000, -127.0000000000000568, -150.2000000000013245 ) ) ;
#5455=CARTESIAN_POINT ( 'NONE',  ( -281.4928932188135491, -127.0000000000000568, 150.2000000000013813 ) ) ;
#5467=EDGE_CURVE ( 'NONE', #3608, #14489, #10913, .T. ) ;
#5468=ORIENTED_EDGE ( 'NONE', *, *, #10154, .T. ) ;
#5471=EDGE_CURVE ( 'NONE', #14489, #4595, #5323, .T. ) ;
#5475=ORIENTED_EDGE ( 'NONE', *, *, #7252, .T. ) ;
#5480=FACE_OUTER_BOUND ( 'NONE', #14359, .T. ) ;
#5486=CARTESIAN_POINT ( 'NONE',  ( -7.703011046602857601E-15, -132.2000000000000455, 0.000000000000000000 ) ) ;
#5490=CARTESIAN_POINT ( 'NONE',  ( -283.2140793454688605, 271.9822575857424454, 145.6220388411722695 ) ) ;
#5491=ADVANCED_FACE ( 'NONE', ( #12969 ), #1804, .F. ) ;
#5503=DIRECTION ( 'NONE',  ( 0.000000000000000000, -1.000000000000000000, -3.495664435217746987E-15 ) ) ;
#5509=EDGE_LOOP ( 'NONE', ( #9912, #9444, #8670, #2860 ) ) ;
#5511=DIRECTION ( 'NONE',  ( 0.000000000000000000, 0.000000000000000000, 1.000000000000000000 ) ) ;
#5517=ORIENTED_EDGE ( 'NONE', *, *, #4417, .F. ) ;
#5518=CARTESIAN_POINT ( 'NONE',  ( 280.8708543776410806, 270.9956429438695409, 149.1582675804705218 ) ) ;
#5528=ORIENTED_EDGE ( 'NONE', *, *, #17271, .T. ) ;
#5529=ADVANCED_FACE ( 'NONE', ( #23670 ), #22086, .F. ) ;
#5534=DIRECTION ( 'NONE',  ( 1.000000000000000000, 0.000000000000000000, 0.000000000000000000 ) ) ;
#5546=CARTESIAN_POINT ( 'NONE',  ( -280.0000000000000568, 267.7999999999999545, -150.1999999999999318 ) ) ;
#5548=ORIENTED_EDGE ( 'NONE', *, *, #5129, .F. ) ;
#5550=EDGE_CURVE ( 'NONE', #23104, #2171, #6164, .T. ) ;
#5551=AXIS2_PLACEMENT_3D ( 'NONE', #11444, #12648, #5743 ) ;
#5560=DIRECTION ( 'NONE',  ( -0.000000000000000000, 1.000000000000000000, -0.000000000000000000 ) ) ;
#5562=CARTESIAN_POINT ( 'NONE',  ( 284.2295083325149108, 270.8299054689547347, 145.9020829022174439 ) ) ;
#5574=CARTESIAN_POINT ( 'NONE',  ( 281.2440776823445390, 268.3758453455904487, -147.1427398886702349 ) ) ;
#5577=CARTESIAN_POINT ( 'NONE',  ( 0.000000000000000000, -127.0000000000000568, 150.2000000000013813 ) ) ;
#5582=EDGE_CURVE ( 'NONE', #1647, #9091, #12744, .T. ) ;
#5584=EDGE_CURVE ( 'NONE', #12385, #5390, #9074, .T. ) ;
#5591=CARTESIAN_POINT ( 'NONE',  ( -280.6228333615952693, 271.9320353020572156, 148.1755088701073930 ) ) ;
#5592=EDGE_CURVE ( 'NONE', #2171, #22539, #16216, .T. ) ;
#5599=EDGE_CURVE ( 'NONE', #16083, #4595, #12619, .T. ) ;
#5602=AXIS2_PLACEMENT_3D ( 'NONE', #9765, #7705, #17121 ) ;
#5604=ORIENTED_EDGE ( 'NONE', *, *, #171, .T. ) ;
#5608=AXIS2_PLACEMENT_3D ( 'NONE', #15593, #21480, #19666 ) ;
#5611=CARTESIAN_POINT ( 'NONE',  ( -312.2000000000014666, -129.2000000000000455, -146.4928932188134070 ) ) ;
#5627=DIRECTION ( 'NONE',  ( 0.000000000000000000, 0.000000000000000000, 1.000000000000000000 ) ) ;
#5628=CARTESIAN_POINT ( 'NONE',  ( -287.4000000000014552, -127.0000000000000568, 146.4928932188134638 ) ) ;
#5634=EDGE_LOOP ( 'NONE', ( #5548, #20199 ) ) ;
#5638=ORIENTED_EDGE ( 'NONE', *, *, #13754, .F. ) ;
#5652=CARTESIAN_POINT ( 'NONE',  ( 281.3689414351989626, 272.8938770989752811, -145.2488155364688680 ) ) ;
#5657=CARTESIAN_POINT ( 'NONE',  ( 281.2440776823444253, 268.3758453455903918, 147.1427398886702917 ) ) ;
#5667=DIRECTION ( 'NONE',  ( 0.000000000000000000, -0.000000000000000000, 1.000000000000000000 ) ) ;
#5668=LINE ( 'NONE', #9421, #6827 ) ;
#5670=CIRCLE ( 'NONE', #23794, 2.199999999999979750 ) ;
#5675=EDGE_LOOP ( 'NONE', ( #3318, #9562, #8182, #2909 ) ) ;
#5677=DIRECTION ( 'NONE',  ( -1.000000000000000000, -0.000000000000000000, -0.000000000000000000 ) ) ;
#5680=CARTESIAN_POINT ( 'NONE',  ( 284.1268706878666990, 270.9682701916306087, 145.8706349181169628 ) ) ;
#5694=CARTESIAN_POINT ( 'NONE',  ( 280.2488155364688396, 272.8938770989753948, -146.3689414351990195 ) ) ;
#5697=VERTEX_POINT ( 'NONE', #11643 ) ;
#5699=CARTESIAN_POINT ( 'NONE',  ( 284.1320353020572611, 270.9755088701073191, -145.8700598572183651 ) ) ;
#5705=DIRECTION ( 'NONE',  ( 0.000000000000000000, -1.000000000000000000, 0.000000000000000000 ) ) ;
#5712=FACE_OUTER_BOUND ( 'NONE', #5288, .T. ) ;
#5713=CARTESIAN_POINT ( 'NONE',  ( -281.2440776823445390, 269.1610889986682764, -150.0646579186752092 ) ) ;
#5725=CARTESIAN_POINT ( 'NONE',  ( 281.0927021017106426, 269.6958543268121957, 145.4976310729378497 ) ) ;
#5739=STYLED_ITEM ( 'NONE', ( #7983 ), #9029 ) ;
#5743=DIRECTION ( 'NONE',  ( 0.000000000000000000, -1.000000000000000000, 0.000000000000000000 ) ) ;
#5751=DIRECTION ( 'NONE',  ( 1.000000000000000000, 0.000000000000000000, 0.000000000000000000 ) ) ;
#5760=ADVANCED_FACE ( 'NONE', ( #2041 ), #9432, .F. ) ;
#5766=EDGE_CURVE ( 'NONE', #3355, #2544, #17057, .T. ) ;
#5769=CARTESIAN_POINT ( 'NONE',  ( -285.2000000000000455, 267.7999999999999545, 0.000000000000000000 ) ) ;
#5772=EDGE_CURVE ( 'NONE', #7386, #8023, #12119, .T. ) ;
#5785=PRODUCT_CONTEXT ( 'NONE', #1505, 'mechanical' ) ;
#5794=ORIENTED_EDGE ( 'NONE', *, *, #14090, .T. ) ;
#5795=VERTEX_POINT ( 'NONE', #4828 ) ;
#5800=DIRECTION ( 'NONE',  ( 0.000000000000000000, 0.000000000000000000, 1.000000000000000000 ) ) ;
#5813=CARTESIAN_POINT ( 'NONE',  ( -280.0000000000000568, 272.9999999999999432, -144.9999999999999716 ) ) ;
#5815=CARTESIAN_POINT ( 'NONE',  ( -281.1045205713626842, 269.7080393212557965, -145.4986342070536978 ) ) ;
#5817=LINE ( 'NONE', #22345, #6126 ) ;
#5822=EDGE_LOOP ( 'NONE', ( #16592, #12037, #16861, #8360, #9617, #19551, #1308, #3794 ) ) ;
#5826=ORIENTED_EDGE ( 'NONE', *, *, #11717, .F. ) ;
#5829=ORIENTED_EDGE ( 'NONE', *, *, #185, .T. ) ;
#5832=CARTESIAN_POINT ( 'NONE',  ( -40.00000000000000000, 100.0000000000000000, 150.2000000000009550 ) ) ;
#5834=ADVANCED_FACE ( 'NONE', ( #6398 ), #23046, .T. ) ;
#5837=CARTESIAN_POINT ( 'NONE',  ( -280.1247002395581376, 272.9663407402831012, 145.6822561791009321 ) ) ;
#5842=CARTESIAN_POINT ( 'NONE',  ( -281.4928932188134354, 267.7999999999999545, -150.2299999999999329 ) ) ;
#5847=CARTESIAN_POINT ( 'NONE',  ( 284.5699028110927316, 270.4339272673396977, 145.9952621458756710 ) ) ;
#5850=ADVANCED_FACE ( 'NONE', ( #10280 ), #19676, .F. ) ;
#5855=ORIENTED_EDGE ( 'NONE', *, *, #14840, .F. ) ;
#5883=CARTESIAN_POINT ( 'NONE',  ( 281.0570750465942638, 270.1062614524586820, 149.6728700860325318 ) ) ;
#5888=CARTESIAN_POINT ( 'NONE',  ( 281.0927021017106426, 269.6958543268121957, -145.4976310729377644 ) ) ;
#5891=FACE_BOUND ( 'NONE', #10859, .T. ) ;
#5896=ORIENTED_EDGE ( 'NONE', *, *, #20806, .T. ) ;
#5901=CIRCLE ( 'NONE', #2810, 5.249999999999973355 ) ;
#5905=CARTESIAN_POINT ( 'NONE',  ( -285.2000000000012960, -74.99999999999899103, 90.00000000000000000 ) ) ;
#5909=ORIENTED_EDGE ( 'NONE', *, *, #14633, .T. ) ;
#5913=CARTESIAN_POINT ( 'NONE',  ( -280.0627246244602020, 273.0000000000000568, -145.3431883566700549 ) ) ;
#5932=CARTESIAN_POINT ( 'NONE',  ( 280.1244295015775378, 273.0299999999999727, -145.6847249064869061 ) ) ;
#5933=EDGE_CURVE ( 'NONE', #23782, #14990, #416, .T. ) ;
#5934=ORIENTED_EDGE ( 'NONE', *, *, #19297, .T. ) ;
#5935=AXIS2_PLACEMENT_3D ( 'NONE', #7351, #1427, #12483 ) ;
#5941=DIRECTION ( 'NONE',  ( -1.000000000000000000, 0.000000000000000000, 0.000000000000000000 ) ) ;
#5945=ORIENTED_EDGE ( 'NONE', *, *, #19719, .T. ) ;
#5953=CARTESIAN_POINT ( 'NONE',  ( -280.0000000000000000, 273.0299999999999727, -144.9999999999999716 ) ) ;
#5959=CARTESIAN_POINT ( 'NONE',  ( 281.4928932188134354, -127.0000000000000568, -152.4000000000012847 ) ) ;
#5962=CARTESIAN_POINT ( 'NONE',  ( 280.6807971656550080, 272.9999999999999432, 145.1244294735509470 ) ) ;
#5966=AXIS2_PLACEMENT_3D ( 'NONE', #18997, #8031, #17332 ) ;
#5967=DIRECTION ( 'NONE',  ( 0.000000000000000000, -1.000000000000000000, 0.000000000000000000 ) ) ;
#5986=DIRECTION ( 'NONE',  ( 3.495664435217746987E-15, -1.000000000000000000, 0.000000000000000000 ) ) ;
#5989=ORIENTED_EDGE ( 'NONE', *, *, #11895, .F. ) ;
#6018=DIRECTION ( 'NONE',  ( -1.000000000000000000, 0.000000000000000000, 0.000000000000000000 ) ) ;
#6021=ADVANCED_FACE ( 'NONE', ( #9659 ), #16764, .T. ) ;
#6024=CARTESIAN_POINT ( 'NONE',  ( -288.2000000000013529, -89.99999999999896261, -40.33333333333332860 ) ) ;
#6025=ORIENTED_EDGE ( 'NONE', *, *, #10406, .F. ) ;
#6027=ADVANCED_FACE ( 'NONE', ( #584, #5891, #11254, #18671, #11614, #7951, #20734, #15210, #4195, #13065 ), #15329, .T. ) ;
#6039=LINE ( 'NONE', #15489, #9620 ) ;
#6041=CARTESIAN_POINT ( 'NONE',  ( 279.9999999999999432, -127.0000000000000568, 147.2000000000013813 ) ) ;
#6045=CARTESIAN_POINT ( 'NONE',  ( -282.2000000000007276, 75.00000000000099476, -90.00000000000000000 ) ) ;
#6047=CARTESIAN_POINT ( 'NONE',  ( 281.3684665762324926, 268.0840560642351988, -147.1696999999999207 ) ) ;
#6054=CARTESIAN_POINT ( 'NONE',  ( 281.6795879751484222, 272.7329465209282375, -145.3118087683467934 ) ) ;
#6066=AXIS2_PLACEMENT_3D ( 'NONE', #18558, #7454, #2011 ) ;
#6069=DIRECTION ( 'NONE',  ( -1.000000000000000000, -0.000000000000000000, -0.000000000000000000 ) ) ;
#6071=CARTESIAN_POINT ( 'NONE',  ( -282.1854425596108058, 268.0906609804448522, 146.3673129565597719 ) ) ;
#6082=ORIENTED_EDGE ( 'NONE', *, *, #13829, .F. ) ;
#6090=DIRECTION ( 'NONE',  ( 6.640089860198304064E-16, 1.000000000000000000, -4.183096374613631247E-18 ) ) ;
#6111=AXIS2_PLACEMENT_3D ( 'NONE', #15559, #10352, #8537 ) ;
#6115=ORIENTED_EDGE ( 'NONE', *, *, #10546, .F. ) ;
#6120=AXIS2_PLACEMENT_3D ( 'NONE', #12327, #15801, #17837 ) ;
#6122=AXIS2_PLACEMENT_3D ( 'NONE', #16494, #21919, #16740 ) ;
#6124=LINE ( 'NONE', #6252, #2781 ) ;
#6126=VECTOR ( 'NONE', #14760, 1000.000000000000000 ) ;
#6128=ORIENTED_EDGE ( 'NONE', *, *, #1350, .T. ) ;
#6129=CARTESIAN_POINT ( 'NONE',  ( 280.8700598572182798, 270.9755088701073191, 149.1320353020572611 ) ) ;
#6134=LINE ( 'NONE', #19036, #331 ) ;
#6138=DIRECTION ( 'NONE',  ( -1.000000000000000000, 6.640089860198304064E-16, 0.000000000000000000 ) ) ;
#6140=EDGE_LOOP ( 'NONE', ( #2313, #6561, #10537, #21264 ) ) ;
#6154=EDGE_CURVE ( 'NONE', #2180, #19505, #14125, .T. ) ;
#6157=AXIS2_PLACEMENT_3D ( 'NONE', #7354, #16527, #11123 ) ;
#6161=ORIENTED_EDGE ( 'NONE', *, *, #11656, .F. ) ;
#6164=CIRCLE ( 'NONE', #21602, 2.649999999999971934 ) ;
#6166=AXIS2_PLACEMENT_3D ( 'NONE', #22051, #8492, #5162 ) ;
#6186=EDGE_LOOP ( 'NONE', ( #5177, #18357, #16047, #19165 ) ) ;
#6189=EDGE_LOOP ( 'NONE', ( #10646, #18661, #8224, #5375 ) ) ;
#6193=ADVANCED_FACE ( 'NONE', ( #3102 ), #10374, .F. ) ;
#6201=CARTESIAN_POINT ( 'NONE',  ( -281.9771302778489712, 268.7755403010746704, 146.0571734979477014 ) ) ;
#6210=EDGE_CURVE ( 'NONE', #67, #10559, #1926, .T. ) ;
#6211=CARTESIAN_POINT ( 'NONE',  ( 283.1956429438695295, 271.9582675804705332, 145.6220388411722979 ) ) ;
#6212=CARTESIAN_POINT ( 'NONE',  ( -284.1822575857425477, 271.0140793454687582, -145.8708543776411375 ) ) ;
#6217=PLANE ( 'NONE',  #10619 ) ;
#6222=ORIENTED_EDGE ( 'NONE', *, *, #16485, .T. ) ;
#6247=EDGE_CURVE ( 'NONE', #12957, #1216, #10734, .T. ) ;
#6249=LINE ( 'NONE', #14109, #9838 ) ;
#6252=CARTESIAN_POINT ( 'NONE',  ( -282.2000000000001023, 267.7999999999999545, -146.4928932188134354 ) ) ;
#6255=CARTESIAN_POINT ( 'NONE',  ( 280.3118087683465660, 272.7329465209280670, 146.6795879751483369 ) ) ;
#6259=CARTESIAN_POINT ( 'NONE',  ( 281.7592670532758916, 269.1520027839447948, -145.8708543776411091 ) ) ;
#6270=ADVANCED_FACE ( 'NONE', ( #14706, #14576, #22043, #23386 ), #16036, .T. ) ;
#6273=ADVANCED_FACE ( 'NONE', ( #14246 ), #1531, .F. ) ;
#6286=LINE ( 'NONE', #17407, #15426 ) ;
#6299=VECTOR ( 'NONE', #21540, 1000.000000000000000 ) ;
#6300=CARTESIAN_POINT ( 'NONE',  ( -281.4928932188135491, 267.7999999999999545, 150.1999999999999886 ) ) ;
#6320=EDGE_LOOP ( 'NONE', ( #12613, #14724, #19571, #19035 ) ) ;
#6332=CARTESIAN_POINT ( 'NONE',  ( -285.2000000000014666, -132.2000000000000455, -146.4928932188134070 ) ) ;
#6338=AXIS2_PLACEMENT_3D ( 'NONE', #18806, #11265, #2028 ) ;
#6359=EDGE_CURVE ( 'NONE', #12563, #21417, #1640, .T. ) ;
#6365=EDGE_CURVE ( 'NONE', #2692, #14837, #9138, .T. ) ;
#6381=CARTESIAN_POINT ( 'NONE',  ( 282.1999999999999886, 267.7999999999999545, 146.4928932188134922 ) ) ;
#6385=CARTESIAN_POINT ( 'NONE',  ( 280.8708543776410806, 271.0140793454687582, 149.1822575857424624 ) ) ;
#6391=ORIENTED_EDGE ( 'NONE', *, *, #5599, .T. ) ;
#6393=CARTESIAN_POINT ( 'NONE',  ( 0.000000000000000000, 272.9999999999999432, 3.330669073875469621E-16 ) ) ;
#6394=ORIENTED_EDGE ( 'NONE', *, *, #5129, .T. ) ;
#6398=FACE_OUTER_BOUND ( 'NONE', #5072, .T. ) ;
#6403=DIRECTION ( 'NONE',  ( 0.000000000000000000, 0.000000000000000000, 1.000000000000000000 ) ) ;
#6410=ORIENTED_EDGE ( 'NONE', *, *, #15714, .F. ) ;
#6414=DIRECTION ( 'NONE',  ( 0.000000000000000000, 0.000000000000000000, 1.000000000000000000 ) ) ;
#6418=CARTESIAN_POINT ( 'NONE',  ( -281.4928932188135491, 267.7999999999999545, 147.1999999999999886 ) ) ;
#6422=CARTESIAN_POINT ( 'NONE',  ( 282.2000000000008981, 9.787860418609723716E-13, 0.000000000000000000 ) ) ;
#6438=VECTOR ( 'NONE', #3846, 1000.000000000000000 ) ;
#6442=LINE ( 'NONE', #775, #14262 ) ;
#6443=CARTESIAN_POINT ( 'NONE',  ( 279.9999999999999432, 272.9999999999999432, -144.9999999999999716 ) ) ;
#6447=DIRECTION ( 'NONE',  ( 1.000000000000000000, -0.000000000000000000, -0.000000000000000000 ) ) ;
#6448=ORIENTED_EDGE ( 'NONE', *, *, #4596, .F. ) ;
#6452=FACE_OUTER_BOUND ( 'NONE', #10949, .T. ) ;
#6453=ORIENTED_EDGE ( 'NONE', *, *, #8341, .T. ) ;
#6463=CARTESIAN_POINT ( 'NONE',  ( -285.2000000000006708, 90.00000000000100897, 37.64999999999996305 ) ) ;
#6467=ORIENTED_EDGE ( 'NONE', *, *, #16661, .F. ) ;
#6472=DIRECTION ( 'NONE',  ( 0.000000000000000000, -1.000000000000000000, 0.000000000000000000 ) ) ;
#6488=CARTESIAN_POINT ( 'NONE',  ( -282.2000000000013529, -89.99999999999897682, 26.98333333333330231 ) ) ;
#6492=CARTESIAN_POINT ( 'NONE',  ( 281.4928932188133217, 267.7999999999999545, 147.1999999999999886 ) ) ;
#6501=CIRCLE ( 'NONE', #16174, 5.249999999999949374 ) ;
#6516=CARTESIAN_POINT ( 'NONE',  ( 0.000000000000000000, -132.2000000000000455, -7.703011046602857601E-15 ) ) ;
#6518=VECTOR ( 'NONE', #2107, 1000.000000000000000 ) ;
#6522=AXIS2_PLACEMENT_3D ( 'NONE', #5832, #22722, #15021 ) ;
#6532=DIRECTION ( 'NONE',  ( 0.000000000000000000, -3.495664435217746987E-15, 1.000000000000000000 ) ) ;
#6535=VECTOR ( 'NONE', #7741, 1000.000000000000000 ) ;
#6536=EDGE_LOOP ( 'NONE', ( #10791, #14486, #23778, #16397 ) ) ;
#6539=ADVANCED_FACE ( 'NONE', ( #20335 ), #3798, .F. ) ;
#6547=CARTESIAN_POINT ( 'NONE',  ( -280.0000000000000568, 272.9999999999999432, 145.0000000000000284 ) ) ;
#6561=ORIENTED_EDGE ( 'NONE', *, *, #2547, .F. ) ;
#6574=EDGE_CURVE ( 'NONE', #7513, #10936, #6905, .T. ) ;
#6581=VECTOR ( 'NONE', #21169, 1000.000000000000000 ) ;
#6586=ORIENTED_EDGE ( 'NONE', *, *, #11316, .T. ) ;
#6589=CARTESIAN_POINT ( 'NONE',  ( -282.2000000000008981, 35.00000000000100897, 102.3500000000000227 ) ) ;
#6590=CARTESIAN_POINT ( 'NONE',  ( 281.4538215477169842, 269.4574776399289249, 145.6842353883612304 ) ) ;
#6605=EDGE_CURVE ( 'NONE', #12563, #13397, #12396, .T. ) ;
#6619=LINE ( 'NONE', #8665, #21134 ) ;
#6621=CARTESIAN_POINT ( 'NONE',  ( -280.3431883566701686, 273.0000000000000568, 145.0627246244602304 ) ) ;
#6624=CARTESIAN_POINT ( 'NONE',  ( -280.4974534559950712, 269.7094021484634823, -146.1021437883072167 ) ) ;
#6625=CARTESIAN_POINT ( 'NONE',  ( 280.8703180930666576, 269.1429506979392272, 146.7484459290826635 ) ) ;
#6628=ORIENTED_EDGE ( 'NONE', *, *, #19934, .F. ) ;
#6629=FACE_OUTER_BOUND ( 'NONE', #15566, .T. ) ;
#6642=CARTESIAN_POINT ( 'NONE',  ( -285.2000000000012960, -74.99999999999899103, -90.00000000000000000 ) ) ;
#6653=FACE_OUTER_BOUND ( 'NONE', #5122, .T. ) ;
#6655=DIRECTION ( 'NONE',  ( 0.000000000000000000, -1.000000000000000000, 0.000000000000000000 ) ) ;
#6667=DIRECTION ( 'NONE',  ( 0.000000000000000000, -0.000000000000000000, 1.000000000000000000 ) ) ;
#6676=ORIENTED_EDGE ( 'NONE', *, *, #734, .T. ) ;
#6678=CARTESIAN_POINT ( 'NONE',  ( 0.000000000000000000, -129.2000000000000455, 7.690461757479017101E-15 ) ) ;
#6698=AXIS2_PLACEMENT_3D ( 'NONE', #15481, #17272, #838 ) ;
#6703=CARTESIAN_POINT ( 'NONE',  ( 281.1045205713626274, 269.7080393212557397, 145.4986342070537546 ) ) ;
#6705=CARTESIAN_POINT ( 'NONE',  ( -285.2000000000013529, -89.99999999999896261, -40.33333333333332860 ) ) ;
#6706=DIRECTION ( 'NONE',  ( -0.000000000000000000, 6.982962677686266711E-15, -1.000000000000000000 ) ) ;
#6711=ORIENTED_EDGE ( 'NONE', *, *, #16941, .T. ) ;
#6716=VECTOR ( 'NONE', #9768, 1000.000000000000000 ) ;
#6726=ORIENTED_EDGE ( 'NONE', *, *, #17526, .F. ) ;
#6749=CIRCLE ( 'NONE', #8688, 35.00000000000000711 ) ;
#6767=EDGE_CURVE ( 'NONE', #4045, #2262, #7135, .T. ) ;
#6775=ORIENTED_EDGE ( 'NONE', *, *, #13795, .F. ) ;
#6780=EDGE_LOOP ( 'NONE', ( #12149, #17615 ) ) ;
#6783=CARTESIAN_POINT ( 'NONE',  ( -280.2497115627123776, 269.9290760626064980, 145.5724317483736741 ) ) ;
#6795=VECTOR ( 'NONE', #16451, 1000.000000000000000 ) ;
#6800=CARTESIAN_POINT ( 'NONE',  ( -281.3333820183296439, 269.5350371479512432, -145.6220388411722126 ) ) ;
#6801=ORIENTED_EDGE ( 'NONE', *, *, #577, .F. ) ;
#6803=EDGE_CURVE ( 'NONE', #16727, #17822, #386, .T. ) ;
#6814=CARTESIAN_POINT ( 'NONE',  ( 281.4928932188134354, -127.0000000000000568, -150.2000000000013245 ) ) ;
#6824=ORIENTED_EDGE ( 'NONE', *, *, #23212, .F. ) ;
#6827=VECTOR ( 'NONE', #9675, 1000.000000000000000 ) ;
#6828=CARTESIAN_POINT ( 'NONE',  ( -281.7350371479513456, 269.1333820183295416, 145.8708543776411659 ) ) ;
#6833=CARTESIAN_POINT ( 'NONE',  ( -282.3062614524588412, 272.4728700860325716, -145.4358181722190579 ) ) ;
#6854=VERTEX_POINT ( 'NONE', #11508 ) ;
#6858=EDGE_LOOP ( 'NONE', ( #8619, #11601 ) ) ;
#6859=CARTESIAN_POINT ( 'NONE',  ( 281.3684665479254932, 268.0880230824753312, 147.1999999999999886 ) ) ;
#6869=LINE ( 'NONE', #22395, #4046 ) ;
#6870=CARTESIAN_POINT ( 'NONE',  ( -285.2000000000006708, 90.00000000000100897, 32.35000000000001563 ) ) ;
#6875=DIRECTION ( 'NONE',  ( 0.000000000000000000, 0.000000000000000000, 1.000000000000000000 ) ) ;
#6876=CARTESIAN_POINT ( 'NONE',  ( -282.2000000000011255, -29.99999999999898037, -105.0000000000000000 ) ) ;
#6877=LINE ( 'NONE', #23182, #4356 ) ;
#6879=DIRECTION ( 'NONE',  ( 0.000000000000000000, -1.000000000000000000, 0.000000000000000000 ) ) ;
#6887=ORIENTED_EDGE ( 'NONE', *, *, #8978, .T. ) ;
#6898=EDGE_LOOP ( 'NONE', ( #20536, #8142, #6801, #8759 ) ) ;
#6901=DIRECTION ( 'NONE',  ( 0.000000000000000000, -3.495664435217746987E-15, 1.000000000000000000 ) ) ;
#6904=FACE_OUTER_BOUND ( 'NONE', #15849, .T. ) ;
#6905=LINE ( 'NONE', #2473, #20784 ) ;
#6911=VECTOR ( 'NONE', #16848, 1000.000000000000000 ) ;
#6913=VECTOR ( 'NONE', #14898, 1000.000000000000000 ) ;
#6921=CYLINDRICAL_SURFACE ( 'NONE', #16987, 5.249999999999942268 ) ;
#6927=EDGE_CURVE ( 'NONE', #2147, #9524, #20246, .T. ) ;
#6929=CARTESIAN_POINT ( 'NONE',  ( -312.2000000000014666, -129.2000000000000455, 146.4928932188134638 ) ) ;
#6961=CARTESIAN_POINT ( 'NONE',  ( -280.2880230824753198, 269.9999999999999432, 145.1244266708878570 ) ) ;
#6974=DIRECTION ( 'NONE',  ( -0.000000000000000000, 1.000000000000000000, 0.000000000000000000 ) ) ;
#6984=VERTEX_POINT ( 'NONE', #21946 ) ;
#6985=CARTESIAN_POINT ( 'NONE',  ( -280.1255313583546354, 269.9999999999999432, -145.2905802150185366 ) ) ;
#6992=CARTESIAN_POINT ( 'NONE',  ( 280.9952621458755289, 268.8927021017106540, 146.8958543268122128 ) ) ;
#6995=CARTESIAN_POINT ( 'NONE',  ( -282.2000000000008981, 35.00000000000100897, 107.6499999999999631 ) ) ;
#7009=EDGE_CURVE ( 'NONE', #12385, #6984, #10006, .T. ) ;
#7016=DIRECTION ( 'NONE',  ( -0.000000000000000000, -1.000000000000000000, -1.110223024625156540E-16 ) ) ;
#7019=ORIENTED_EDGE ( 'NONE', *, *, #16533, .F. ) ;
#7022=DIRECTION ( 'NONE',  ( -1.000000000000000000, -0.000000000000000000, -0.000000000000000000 ) ) ;
#7037=DIRECTION ( 'NONE',  ( 1.000000000000000000, 0.000000000000000000, 0.000000000000000000 ) ) ;
#7046=DIRECTION ( 'NONE',  ( 0.000000000000000000, -0.000000000000000000, 1.000000000000000000 ) ) ;
#7055=EDGE_CURVE ( 'NONE', #21142, #10685, #6124, .T. ) ;
#7065=CARTESIAN_POINT ( 'NONE',  ( -282.2000000000000455, 267.7999999999999545, 146.4928932188134354 ) ) ;
#7071=ORIENTED_EDGE ( 'NONE', *, *, #2571, .T. ) ;
#7078=CARTESIAN_POINT ( 'NONE',  ( 99.99999999999987210, -132.2000000000001023, 152.4000000000014268 ) ) ;
#7091=PRODUCT_DEFINITION_SHAPE ( 'NONE', 'NONE',  #2813 ) ;
#7110=CARTESIAN_POINT ( 'NONE',  ( 284.1582675804705218, 270.9956429438695409, -145.8708543776411091 ) ) ;
#7128=ADVANCED_FACE ( 'NONE', ( #4315 ), #955, .F. ) ;
#7134=DIRECTION ( 'NONE',  ( -6.938893903907227392E-16, -1.000000000000000000, 0.000000000000000000 ) ) ;
#7135=LINE ( 'NONE', #18239, #18220 ) ;
#7141=ORIENTED_EDGE ( 'NONE', *, *, #4932, .F. ) ;
#7148=DIRECTION ( 'NONE',  ( 0.000000000000000000, 0.000000000000000000, 1.000000000000000000 ) ) ;
#7159=LINE ( 'NONE', #3417, #6299 ) ;
#7163=FACE_OUTER_BOUND ( 'NONE', #2890, .T. ) ;
#7168=CARTESIAN_POINT ( 'NONE',  ( -100.0000000000001137, -127.0000000000000853, 147.2000000000013529 ) ) ;
#7170=CARTESIAN_POINT ( 'NONE',  ( 279.9999999999999432, 269.9999999999999432, -144.9999999999999716 ) ) ;
#7171=CARTESIAN_POINT ( 'NONE',  ( -282.2000000000008981, 35.00000000000100897, 105.0000000000000000 ) ) ;
#7173=CARTESIAN_POINT ( 'NONE',  ( -285.0646579186753797, 269.1610889986682196, 146.2440776823445105 ) ) ;
#7175=CARTESIAN_POINT ( 'NONE',  ( 280.4975000228325257, 272.3132312761074445, -147.6054396500289556 ) ) ;
#7177=CARTESIAN_POINT ( 'NONE',  ( -280.0000000000000568, 272.9999999999999432, -144.9999999999999716 ) ) ;
#7179=ADVANCED_FACE ( 'NONE', ( #8820 ), #19681, .F. ) ;
#7197=LINE ( 'NONE', #21816, #4630 ) ;
#7199=CYLINDRICAL_SURFACE ( 'NONE', #355, 5.199999999999982414 ) ;
#7202=CIRCLE ( 'NONE', #13427, 2.649999999999971934 ) ;
#7203=CARTESIAN_POINT ( 'NONE',  ( 279.9999999999999432, 269.9696999999999889, 145.0000000000000284 ) ) ;
#7206=CARTESIAN_POINT ( 'NONE',  ( 0.000000000000000000, 0.000000000000000000, -147.2000000000008981 ) ) ;
#7211=EDGE_CURVE ( 'NONE', #15403, #12940, #6877, .T. ) ;
#7212=DIRECTION ( 'NONE',  ( -6.640089860198304064E-16, -1.000000000000000000, 0.000000000000000000 ) ) ;
#7218=FACE_OUTER_BOUND ( 'NONE', #21928, .T. ) ;
#7225=CARTESIAN_POINT ( 'NONE',  ( -285.2000000000013529, -89.99999999999897682, 24.33333333333333215 ) ) ;
#7240=ORIENTED_EDGE ( 'NONE', *, *, #12890, .T. ) ;
#7252=EDGE_CURVE ( 'NONE', #18466, #22116, #19543, .T. ) ;
#7253=DIRECTION ( 'NONE',  ( 1.000000000000000000, -0.000000000000000000, 0.000000000000000000 ) ) ;
#7265=CIRCLE ( 'NONE', #10007, 35.00000000000000711 ) ;
#7270=LINE ( 'NONE', #3632, #1887 ) ;
#7290=VECTOR ( 'NONE', #4687, 1000.000000000000000 ) ;
#7293=ORIENTED_EDGE ( 'NONE', *, *, #2571, .F. ) ;
#7303=CARTESIAN_POINT ( 'NONE',  ( -281.3689414351990763, 272.8938770989752811, 145.2488155364689248 ) ) ;
#7306=DIRECTION ( 'NONE',  ( 0.000000000000000000, 0.000000000000000000, 1.000000000000000000 ) ) ;
#7321=DIRECTION ( 'NONE',  ( 0.000000000000000000, 0.000000000000000000, -1.000000000000000000 ) ) ;
#7322=CARTESIAN_POINT ( 'NONE',  ( -45.24999999999994316, 100.0000000000000000, 147.2000000000005855 ) ) ;
#7337=LINE ( 'NONE', #9152, #19287 ) ;
#7339=ORIENTED_EDGE ( 'NONE', *, *, #19678, .T. ) ;
#7340=CARTESIAN_POINT ( 'NONE',  ( 280.6220388411721274, 269.5350371479512432, 146.3333820183295586 ) ) ;
#7348=PLANE ( 'NONE',  #7612 ) ;
#7351=CARTESIAN_POINT ( 'NONE',  ( 287.4000000000013415, -127.0000000000000568, -146.4928932188134070 ) ) ;
#7354=CARTESIAN_POINT ( 'NONE',  ( -282.2000000000013529, -89.99999999999897682, 24.33333333333333215 ) ) ;
#7360=CARTESIAN_POINT ( 'NONE',  ( 45.24999999999994316, 100.0000000000000000, -150.2000000000005571 ) ) ;
#7374=CARTESIAN_POINT ( 'NONE',  ( 2.428612866367495853E-14, 35.00000000000002842, 150.2000000000008413 ) ) ;
#7386=VERTEX_POINT ( 'NONE', #7360 ) ;
#7389=CARTESIAN_POINT ( 'NONE',  ( 279.9999999999999432, 269.9697000000000457, -144.9999999999999716 ) ) ;
#7412=CARTESIAN_POINT ( 'NONE',  ( -282.2000000000012960, -74.99999999999899103, -90.00000000000000000 ) ) ;
#7418=DIRECTION ( 'NONE',  ( 1.000000000000000000, -3.495664435217746987E-15, -0.000000000000000000 ) ) ;
#7423=CARTESIAN_POINT ( 'NONE',  ( -281.6810649015078525, 272.7324007871372942, -145.3120962995436116 ) ) ;
#7427=CARTESIAN_POINT ( 'NONE',  ( -285.2000000000010118, 9.892604858775022387E-13, -146.4928932188134070 ) ) ;
#7446=CARTESIAN_POINT ( 'NONE',  ( 280.9755899421581944, 269.7771650631953548, -145.4357337430840289 ) ) ;
#7447=( GEOMETRIC_REPRESENTATION_CONTEXT ( 3 ) GLOBAL_UNCERTAINTY_ASSIGNED_CONTEXT ( ( #10021 ) ) GLOBAL_UNIT_ASSIGNED_CONTEXT ( ( #21885, #10472, #19475 ) ) REPRESENTATION_CONTEXT ( 'NONE', 'WORKASPACE' ) );
#7450=CARTESIAN_POINT ( 'NONE',  ( 281.4928932188134354, -132.2000000000000455, -177.2000000000013529 ) ) ;
#7451=CIRCLE ( 'NONE', #20958, 5.249999999999949374 ) ;
#7452=FACE_OUTER_BOUND ( 'NONE', #20426, .T. ) ;
#7454=DIRECTION ( 'NONE',  ( 1.000000000000000000, -3.495664435217746987E-15, -0.000000000000000000 ) ) ;
#7457=EDGE_LOOP ( 'NONE', ( #2097, #4322, #12967, #20376 ) ) ;
#7458=CARTESIAN_POINT ( 'NONE',  ( 279.9999999999999432, 272.9999999999999432, -144.9999999999999716 ) ) ;
#7465=VECTOR ( 'NONE', #7321, 1000.000000000000000 ) ;
#7466=EDGE_LOOP ( 'NONE', ( #5100, #3745, #4284, #1988 ) ) ;
#7486=ADVANCED_FACE ( 'NONE', ( #16767 ), #17024, .F. ) ;
#7487=CARTESIAN_POINT ( 'NONE',  ( 285.1663417894421855, 268.4816199723479713, 146.3683070494395508 ) ) ;
#7500=CARTESIAN_POINT ( 'NONE',  ( 280.2488155364688396, 269.9132285165673011, -145.5679143846942907 ) ) ;
#7501=VECTOR ( 'NONE', #20752, 1000.000000000000000 ) ;
#7508=LINE ( 'NONE', #50, #9631 ) ;
#7513=VERTEX_POINT ( 'NONE', #13197 ) ;
#7515=CARTESIAN_POINT ( 'NONE',  ( -282.2000000000006708, 90.00000000000100897, 32.35000000000001563 ) ) ;
#7521=CARTESIAN_POINT ( 'NONE',  ( -281.4928932188135491, -129.2000000000000455, 152.4000000000014268 ) ) ;
#7523=EDGE_CURVE ( 'NONE', #16083, #7513, #20990, .T. ) ;
#7528=ORIENTED_EDGE ( 'NONE', *, *, #9825, .F. ) ;
#7541=EDGE_LOOP ( 'NONE', ( #7815, #2364, #10458, #22414 ) ) ;
#7567=EDGE_CURVE ( 'NONE', #12111, #539, #5090, .T. ) ;
#7569=ORIENTED_EDGE ( 'NONE', *, *, #2025, .F. ) ;
#7573=VERTEX_POINT ( 'NONE', #6488 ) ;
#7578=CARTESIAN_POINT ( 'NONE',  ( 282.6188186979285888, 272.3436892194421262, -145.4976310729377644 ) ) ;
#7596=CARTESIAN_POINT ( 'NONE',  ( -285.2000000000010687, -19.99999999999898392, 105.0000000000000000 ) ) ;
#7597=ORIENTED_EDGE ( 'NONE', *, *, #10081, .F. ) ;
#7601=ORIENTED_EDGE ( 'NONE', *, *, #12482, .F. ) ;
#7603=CARTESIAN_POINT ( 'NONE',  ( 285.1999999999999318, 269.9999999999999432, 146.4928932188134638 ) ) ;
#7606=CARTESIAN_POINT ( 'NONE',  ( 285.0335297745771186, 269.1488036478618824, 146.2439791848364621 ) ) ;
#7607=DIRECTION ( 'NONE',  ( -0.000000000000000000, -0.000000000000000000, 1.000000000000000000 ) ) ;
#7608=DIRECTION ( 'NONE',  ( 1.000000000000000000, 0.000000000000000000, -0.000000000000000000 ) ) ;
#7612=AXIS2_PLACEMENT_3D ( 'NONE', #22063, #9046, #7212 ) ;
#7624=CARTESIAN_POINT ( 'NONE',  ( 284.9324007871372828, 269.4810649015076933, -146.1807969192697385 ) ) ;
#7626=LINE ( 'NONE', #22111, #6913 ) ;
#7627=FACE_OUTER_BOUND ( 'NONE', #1553, .T. ) ;
#7645=CARTESIAN_POINT ( 'NONE',  ( -285.2000000000014666, -127.0000000000000568, -146.4928932188134070 ) ) ;
#7649=DIRECTION ( 'NONE',  ( 0.000000000000000000, 1.000000000000000000, -0.000000000000000000 ) ) ;
#7651=CARTESIAN_POINT ( 'NONE',  ( -281.3689414351990763, 272.8938770989752811, -145.2488155364688396 ) ) ;
#7666=VECTOR ( 'NONE', #5627, 1000.000000000000000 ) ;
#7669=AXIS2_PLACEMENT_3D ( 'NONE', #8666, #17959, #2969 ) ;
#7705=DIRECTION ( 'NONE',  ( 0.000000000000000000, 0.000000000000000000, 1.000000000000000000 ) ) ;
#7724=LINE ( 'NONE', #22434, #20315 ) ;
#7725=CARTESIAN_POINT ( 'NONE',  ( -281.4928932188134354, -127.0000000000000568, -152.4000000000012847 ) ) ;
#7734=VECTOR ( 'NONE', #13179, 1000.000000000000000 ) ;
#7739=ORIENTED_EDGE ( 'NONE', *, *, #22085, .F. ) ;
#7741=DIRECTION ( 'NONE',  ( -1.000000000000000000, -0.000000000000000000, -0.000000000000000000 ) ) ;
#7743=EDGE_CURVE ( 'NONE', #11281, #23782, #1873, .T. ) ;
#7746=CARTESIAN_POINT ( 'NONE',  ( -280.0000000000000000, 270.0000000000000000, -144.9999999999999716 ) ) ;
#7752=FACE_BOUND ( 'NONE', #13351, .T. ) ;
#7754=SURFACE_STYLE_USAGE ( .BOTH. , #621 ) ;
#7758=CARTESIAN_POINT ( 'NONE',  ( 280.6220388411722411, 271.9582675804705900, -148.1956429438695011 ) ) ;
#7772=CARTESIAN_POINT ( 'NONE',  ( -285.2000000000012960, -74.99999999999899103, 90.00000000000000000 ) ) ;
#7774=CARTESIAN_POINT ( 'NONE',  ( -281.4928932188134354, 267.7999999999999545, -147.1999999999999318 ) ) ;
#7777=DIRECTION ( 'NONE',  ( -0.000000000000000000, -0.000000000000000000, 1.000000000000000000 ) ) ;
#7779=CARTESIAN_POINT ( 'NONE',  ( 280.6847249064868492, 273.0299999999999159, 145.1244295015775947 ) ) ;
#7799=CARTESIAN_POINT ( 'NONE',  ( 281.4928932188133217, -127.0000000000000568, 152.4000000000014268 ) ) ;
#7810=AXIS2_PLACEMENT_3D ( 'NONE', #1320, #13808, #8700 ) ;
#7815=ORIENTED_EDGE ( 'NONE', *, *, #460, .F. ) ;
#7825=CARTESIAN_POINT ( 'NONE',  ( 281.7350371479512319, 269.1333820183295416, -145.8708543776411091 ) ) ;
#7831=EDGE_CURVE ( 'NONE', #19104, #21466, #13395, .T. ) ;
#7844=ORIENTED_EDGE ( 'NONE', *, *, #2815, .T. ) ;
#7860=DIRECTION ( 'NONE',  ( -1.000000000000000000, 3.495664435217746987E-15, 0.000000000000000000 ) ) ;
#7889=ORIENTED_EDGE ( 'NONE', *, *, #7523, .F. ) ;
#7890=CARTESIAN_POINT ( 'NONE',  ( -280.2488155364688964, 269.9427398886703031, -145.5758453455903805 ) ) ;
#7893=EDGE_LOOP ( 'NONE', ( #21361, #23648, #20024, #11053 ) ) ;
#7894=AXIS2_PLACEMENT_3D ( 'NONE', #22886, #23244, #6472 ) ;
#7900=ORIENTED_EDGE ( 'NONE', *, *, #12562, .T. ) ;
#7901=DIRECTION ( 'NONE',  ( -0.000000000000000000, -0.000000000000000000, -1.000000000000000000 ) ) ;
#7933=CARTESIAN_POINT ( 'NONE',  ( 281.4533442688713194, 269.4578961534455175, -145.6839617489740988 ) ) ;
#7944=LINE ( 'NONE', #4436, #11558 ) ;
#7945=EDGE_CURVE ( 'NONE', #20948, #22842, #7451, .T. ) ;
#7949=AXIS2_PLACEMENT_3D ( 'NONE', #23465, #21538, #7046 ) ;
#7951=FACE_BOUND ( 'NONE', #19980, .T. ) ;
#7952=CARTESIAN_POINT ( 'NONE',  ( 99.99999999999987210, -132.2000000000003013, -113.4834095219707848 ) ) ;
#7960=EDGE_CURVE ( 'NONE', #2349, #603, #5901, .T. ) ;
#7970=ORIENTED_EDGE ( 'NONE', *, *, #12689, .T. ) ;
#7973=EDGE_CURVE ( 'NONE', #2180, #2544, #22987, .T. ) ;
#7983=PRESENTATION_STYLE_ASSIGNMENT (( #7754 ) ) ;
#7984=EDGE_CURVE ( 'NONE', #14489, #9258, #11824, .T. ) ;
#8012=CARTESIAN_POINT ( 'NONE',  ( -280.0000000000000000, 273.0000000000000000, -144.9999999999999716 ) ) ;
#8021=FACE_OUTER_BOUND ( 'NONE', #6186, .T. ) ;
#8023=VERTEX_POINT ( 'NONE', #12078 ) ;
#8027=CARTESIAN_POINT ( 'NONE',  ( 45.00000000000000000, 269.9999999999999432, 5.249999999999973355 ) ) ;
#8031=DIRECTION ( 'NONE',  ( 0.000000000000000000, -3.495664435217746987E-15, 1.000000000000000000 ) ) ;
#8032=ORIENTED_EDGE ( 'NONE', *, *, #5584, .F. ) ;
#8048=CARTESIAN_POINT ( 'NONE',  ( -281.4928932188134354, -127.0000000000000568, -152.4000000000012847 ) ) ;
#8053=ORIENTED_EDGE ( 'NONE', *, *, #23033, .F. ) ;
#8059=DIRECTION ( 'NONE',  ( -1.000000000000000000, -0.000000000000000000, -0.000000000000000000 ) ) ;
#8063=( GEOMETRIC_REPRESENTATION_CONTEXT ( 3 ) GLOBAL_UNCERTAINTY_ASSIGNED_CONTEXT ( ( #8856 ) ) GLOBAL_UNIT_ASSIGNED_CONTEXT ( ( #11883, #4355, #10060 ) ) REPRESENTATION_CONTEXT ( 'NONE', 'WORKASPACE' ) );
#8083=ORIENTED_EDGE ( 'NONE', *, *, #9177, .F. ) ;
#8091=CIRCLE ( 'NONE', #22333, 5.199999999999982414 ) ;
#8094=B_SPLINE_CURVE_WITH_KNOTS ( 'NONE', 3,
 ( #13447, #13219, #7487, #7606, #20764, #131, #14877, #5562, #5680, #17157, #9800, #4228, #13326, #18949, #12971, #13095, #2412, #614, #20278, #20405 ),
 .UNSPECIFIED., .F., .F.,
 ( 4, 2, 2, 2, 2, 2, 2, 2, 2, 4 ),
 ( 0.000000000000000000, 0.001035985217005892974, 0.002071970434011785947, 0.003107955651017679354, 0.003625948259520565126, 0.004143940868023451331, 0.005179926085029106647, 0.006215911302034762831, 0.007251896519040418147, 0.008287881736046073464 ),
 .UNSPECIFIED. ) ;
#8098=ORIENTED_EDGE ( 'NONE', *, *, #5766, .F. ) ;
#8105=PLANE ( 'NONE',  #6698 ) ;
#8108=ORIENTED_EDGE ( 'NONE', *, *, #16485, .F. ) ;
#8115=DIRECTION ( 'NONE',  ( -0.000000000000000000, -0.000000000000000000, 1.000000000000000000 ) ) ;
#8121=CARTESIAN_POINT ( 'NONE',  ( 287.4000000000013415, -132.2000000000000455, 146.4928932188134638 ) ) ;
#8122=EDGE_CURVE ( 'NONE', #2147, #21880, #22215, .T. ) ;
#8133=CARTESIAN_POINT ( 'NONE',  ( -280.2488155364689533, 272.8646579186752774, 146.3610889986682935 ) ) ;
#8139=LINE ( 'NONE', #17065, #19402 ) ;
#8142=ORIENTED_EDGE ( 'NONE', *, *, #3515, .F. ) ;
#8143=CARTESIAN_POINT ( 'NONE',  ( -280.8708543776411943, 269.1333820183295416, -146.7350371479512887 ) ) ;
#8152=CARTESIAN_POINT ( 'NONE',  ( 281.7592670532758916, 269.1520027839447948, 145.8708543776412228 ) ) ;
#8158=ADVANCED_FACE ( 'NONE', ( #20284 ), #17931, .F. ) ;
#8159=CARTESIAN_POINT ( 'NONE',  ( -285.2000000000006708, 90.00000000000102318, -35.00000000000001421 ) ) ;
#8161=CYLINDRICAL_SURFACE ( 'NONE', #13917, 2.199999999999979750 ) ;
#8163=ORIENTED_EDGE ( 'NONE', *, *, #16430, .T. ) ;
#8170=ORIENTED_EDGE ( 'NONE', *, *, #4635, .T. ) ;
#8182=ORIENTED_EDGE ( 'NONE', *, *, #2311, .T. ) ;
#8211=LINE ( 'NONE', #19301, #11887 ) ;
#8224=ORIENTED_EDGE ( 'NONE', *, *, #4932, .T. ) ;
#8231=CARTESIAN_POINT ( 'NONE',  ( -281.4928932188134354, -132.2000000000000455, -152.4000000000012562 ) ) ;
#8232=EDGE_LOOP ( 'NONE', ( #11664, #23713 ) ) ;
#8238=CARTESIAN_POINT ( 'NONE',  ( -280.1244295015776515, 273.0299999999999159, 145.6847249064869629 ) ) ;
#8259=CARTESIAN_POINT ( 'NONE',  ( -282.6188186979287025, 272.3436892194421262, -145.4976310729377929 ) ) ;
#8263=DIRECTION ( 'NONE',  ( -0.000000000000000000, -1.000000000000000000, -1.110223024625156540E-16 ) ) ;
#8267=DIRECTION ( 'NONE',  ( 0.000000000000000000, -1.000000000000000000, -5.286776307738891306E-15 ) ) ;
#8268=ADVANCED_FACE ( 'NONE', ( #13333 ), #13457, .F. ) ;
#8294=AXIS2_PLACEMENT_3D ( 'NONE', #20831, #4518, #8267 ) ;
#8305=EDGE_LOOP ( 'NONE', ( #16513, #18232, #18710, #7240 ) ) ;
#8306=DIRECTION ( 'NONE',  ( 0.000000000000000000, 0.000000000000000000, -1.000000000000000000 ) ) ;
#8314=DIRECTION ( 'NONE',  ( -1.000000000000000000, 3.495664435217746987E-15, 0.000000000000000000 ) ) ;
#8324=VECTOR ( 'NONE', #13383, 1000.000000000000000 ) ;
#8340=ORIENTED_EDGE ( 'NONE', *, *, #14633, .F. ) ;
#8341=EDGE_CURVE ( 'NONE', #21062, #5386, #17767, .T. ) ;
#8343=CARTESIAN_POINT ( 'NONE',  ( 34.75000000000003553, 100.0000000000000000, 150.2000000000009550 ) ) ;
#8349=VECTOR ( 'NONE', #10605, 1000.000000000000000 ) ;
#8350=CARTESIAN_POINT ( 'NONE',  ( -280.6220388411723548, 271.9582675804705332, 148.1956429438695579 ) ) ;
#8352=VERTEX_POINT ( 'NONE', #19424 ) ;
#8359=LINE ( 'NONE', #11670, #23481 ) ;
#8360=ORIENTED_EDGE ( 'NONE', *, *, #13203, .F. ) ;
#8361=CARTESIAN_POINT ( 'NONE',  ( 312.2000000000013529, -132.2000000000000455, 146.4928932188134638 ) ) ;
#8362=VECTOR ( 'NONE', #18123, 1000.000000000000000 ) ;
#8372=CARTESIAN_POINT ( 'NONE',  ( -280.0000000000000568, 272.9999999999999432, -144.9999999999999716 ) ) ;
#8389=CARTESIAN_POINT ( 'NONE',  ( 282.1433523009092710, 268.3743436287468853, 146.2447782964894714 ) ) ;
#8391=CIRCLE ( 'NONE', #11486, 5.249999999999991118 ) ;
#8399=AXIS2_PLACEMENT_3D ( 'NONE', #10800, #15131, #11392 ) ;
#8407=ADVANCED_FACE ( 'NONE', ( #3140 ), #3363, .F. ) ;
#8428=DIRECTION ( 'NONE',  ( 1.000000000000000000, -6.640089860198304064E-16, -0.000000000000000000 ) ) ;
#8429=CARTESIAN_POINT ( 'NONE',  ( -284.1320353020573179, 270.9755088701073191, 145.8700598572184504 ) ) ;
#8437=EDGE_CURVE ( 'NONE', #11652, #9214, #14945, .T. ) ;
#8441=EDGE_LOOP ( 'NONE', ( #4272, #19522 ) ) ;
#8445=DIRECTION ( 'NONE',  ( 0.000000000000000000, -3.495664435217746987E-15, 1.000000000000000000 ) ) ;
#8453=EDGE_CURVE ( 'NONE', #22988, #18096, #23405, .T. ) ;
#8466=CARTESIAN_POINT ( 'NONE',  ( -285.2000000000007276, 75.00000000000100897, -90.00000000000000000 ) ) ;
#8471=FACE_OUTER_BOUND ( 'NONE', #2288, .T. ) ;
#8476=CARTESIAN_POINT ( 'NONE',  ( 281.4928932188134354, -127.0000000000000568, -150.2000000000013245 ) ) ;
#8481=ORIENTED_EDGE ( 'NONE', *, *, #3534, .F. ) ;
#8489=DIRECTION ( 'NONE',  ( 0.000000000000000000, -3.495664435217746987E-15, -1.000000000000000000 ) ) ;
#8490=PLANE ( 'NONE',  #336 ) ;
#8492=DIRECTION ( 'NONE',  ( -0.000000000000000000, -0.000000000000000000, 1.000000000000000000 ) ) ;
#8494=LINE ( 'NONE', #8361, #22712 ) ;
#8497=AXIS2_PLACEMENT_3D ( 'NONE', #9507, #3926, #22283 ) ;
#8501=FACE_OUTER_BOUND ( 'NONE', #16141, .T. ) ;
#8505=CARTESIAN_POINT ( 'NONE',  ( -284.1582675804706355, 270.9956429438695409, -145.8708543776411375 ) ) ;
#8509=FACE_BOUND ( 'NONE', #10636, .T. ) ;
#8517=DIRECTION ( 'NONE',  ( 1.000000000000000000, 0.000000000000000000, 0.000000000000000000 ) ) ;
#8522=CARTESIAN_POINT ( 'NONE',  ( -281.3683070494395224, 268.4816199723481418, 150.1663417894422423 ) ) ;
#8529=CARTESIAN_POINT ( 'NONE',  ( -281.4928932188134922, 267.7999999999999545, -150.1999999999999602 ) ) ;
#8530=ORIENTED_EDGE ( 'NONE', *, *, #11277, .F. ) ;
#8537=DIRECTION ( 'NONE',  ( 1.000000000000000000, 0.000000000000000000, 0.000000000000000000 ) ) ;
#8541=CARTESIAN_POINT ( 'NONE',  ( -283.4379565153279259, 271.7159870726003987, -145.6846668451111668 ) ) ;
#8542=LINE ( 'NONE', #7177, #381 ) ;
#8548=CARTESIAN_POINT ( 'NONE',  ( 45.24999999999996447, 100.0000000000000000, 150.2000000000009550 ) ) ;
#8558=CARTESIAN_POINT ( 'NONE',  ( -283.9159870726005579, 271.2379565153279373, 145.8082263737022686 ) ) ;
#8559=ORIENTED_EDGE ( 'NONE', *, *, #18460, .T. ) ;
#8561=CARTESIAN_POINT ( 'NONE',  ( -281.3673129565598288, 268.0906609804448522, -147.1854425596106637 ) ) ;
#8562=CARTESIAN_POINT ( 'NONE',  ( -34.75000000000005684, 100.0000000000000000, -147.2000000000005571 ) ) ;
#8569=ORIENTED_EDGE ( 'NONE', *, *, #10441, .F. ) ;
#8579=EDGE_CURVE ( 'NONE', #10559, #17768, #233, .T. ) ;
#8583=ORIENTED_EDGE ( 'NONE', *, *, #22580, .T. ) ;
#8589=ORIENTED_EDGE ( 'NONE', *, *, #313, .T. ) ;
#8598=CARTESIAN_POINT ( 'NONE',  ( -280.3113419039146947, 269.8873946496626104, 145.7095819834011650 ) ) ;
#8599=DIRECTION ( 'NONE',  ( -1.000000000000000000, 0.000000000000000000, -0.000000000000000000 ) ) ;
#8604=ORIENTED_EDGE ( 'NONE', *, *, #59, .F. ) ;
#8610=EDGE_CURVE ( 'NONE', #4025, #12563, #7724, .T. ) ;
#8614=EDGE_CURVE ( 'NONE', #14837, #11842, #13308, .T. ) ;
#8617=CARTESIAN_POINT ( 'NONE',  ( -282.1697000000000912, 268.0840560642353125, -146.3684665762323789 ) ) ;
#8618=AXIS2_PLACEMENT_3D ( 'NONE', #6422, #11667, #9710 ) ;
#8619=ORIENTED_EDGE ( 'NONE', *, *, #4184, .F. ) ;
#8628=DIRECTION ( 'NONE',  ( 1.000000000000000000, 0.000000000000000000, -0.000000000000000000 ) ) ;
#8631=CARTESIAN_POINT ( 'NONE',  ( -281.4928932188135491, 267.7999999999999545, 150.1999999999999886 ) ) ;
#8634=B_SPLINE_SURFACE_WITH_KNOTS ( 'NONE', 1, 3, ( 
 ( #18744, #17079, #20565, #15402, #6212, #13619, #16723, #7651, #9365, #15049 ),
 ( #4016, #2706, #1124, #4642, #8505, #4870, #8259, #13847, #23096, #8372 ),
 ( #2570, #22967, #10316, #21175, #15880, #12055, #15635, #23332, #4745, #15747 ),
 ( #13975, #8617, #23215, #2808, #12274, #6800, #3046, #14190, #15525, #22850 ) ),
 .UNSPECIFIED., .F., .F., .F.,
 ( 2, 1, 1, 2 ),
 ( 4, 2, 2, 2, 4 ),
 ( -0.01000000000000000021, 0.000000000000000000, 1.000000000000000000, 1.010099999999999998 ),
 ( 0.000000000000000000, 0.2500000000000000000, 0.5000000000000000000, 0.7500000000000000000, 1.000000000000000000 ),
 .UNSPECIFIED. ) ;
#8642=CARTESIAN_POINT ( 'NONE',  ( -285.2000000000011255, -29.99999999999898037, -102.3500000000000227 ) ) ;
#8646=CARTESIAN_POINT ( 'NONE',  ( 281.4928932188134354, 267.8000000000000114, -147.1999999999999318 ) ) ;
#8649=CARTESIAN_POINT ( 'NONE',  ( -281.0927021017107563, 269.6958543268121957, 145.4976310729378213 ) ) ;
#8653=CARTESIAN_POINT ( 'NONE',  ( -283.9107452280325106, 271.2314821058793086, -145.8083875057488683 ) ) ;
#8654=VERTEX_POINT ( 'NONE', #15219 ) ;
#8663=CARTESIAN_POINT ( 'NONE',  ( 312.2000000000013529, -132.2000000000000455, 146.4928932188134638 ) ) ;
#8664=LINE ( 'NONE', #21918, #23291 ) ;
#8665=CARTESIAN_POINT ( 'NONE',  ( 7.703011046602857601E-15, -132.2000000000000455, 146.4928932188134638 ) ) ;
#8666=CARTESIAN_POINT ( 'NONE',  ( -285.2000000000013529, -89.99999999999897682, 24.33333333333333215 ) ) ;
#8670=ORIENTED_EDGE ( 'NONE', *, *, #8752, .T. ) ;
#8674=CARTESIAN_POINT ( 'NONE',  ( 281.0571734979477014, 268.7755403010747273, 146.9771302778488860 ) ) ;
#8676=VECTOR ( 'NONE', #18579, 1000.000000000000000 ) ;
#8688=AXIS2_PLACEMENT_3D ( 'NONE', #7206, #8808, #1768 ) ;
#8697=CLOSED_SHELL ( 'NONE', ( #22289, #1948, #16698, #16922, #13730, #14798, #21718, #1303, #6273, #7179, #12342, #13602, #17137, #3406, #19439, #21747, #10137, #21373, #16925, #9635, #14154, #11552, #3048, #458, #2727, #212, #351, #5200, #8845, #21709, #7486, #861, #16541, #10180, #3671, #6027, #1798, #146, #21400, #15637, #13415, #15215, #12634, #6270, #1030, #13428, #19497, #10644, #5834, #18380, #14024, #12503, #5760, #13892, #2040, #10234, #18742, #1130, #23270, #752, #5043, #13970, #13788, #18330, #21288, #481, #23532, #19028, #14047, #10542, #10643, #7128, #9520, #23671, #6021, #2063, #15608, #2302, #5850, #117, #5491, #20397, #2197, #20654, #270, #10915, #11504, #2959, #22015, #6193, #8158, #6539, #20351, #18982, #19866, #21977, #23187, #20492, #19805, #20559, #8268, #8905, #8407, #3002, #23730, #15545, #14014, #14900, #3280, #4066, #15420, #5529 ) ) ;
#8698=CARTESIAN_POINT ( 'NONE',  ( 279.9999999999999432, 267.7999999999999545, 146.4928932188134922 ) ) ;
#8700=DIRECTION ( 'NONE',  ( 4.183096374613631247E-18, 1.000000000000000000, 0.000000000000000000 ) ) ;
#8706=EDGE_CURVE ( 'NONE', #21291, #17822, #8391, .T. ) ;
#8722=CARTESIAN_POINT ( 'NONE',  ( -281.0571594757294065, 268.7755899421580921, 146.9771650631953719 ) ) ;
#8747=CARTESIAN_POINT ( 'NONE',  ( -285.2000000000008981, 35.00000000000100897, 105.0000000000000000 ) ) ;
#8750=ORIENTED_EDGE ( 'NONE', *, *, #84, .T. ) ;
#8752=EDGE_CURVE ( 'NONE', #13397, #16062, #1293, .T. ) ;
#8758=CARTESIAN_POINT ( 'NONE',  ( -281.4301685943534039, 268.1431883566699526, 150.1999999999999602 ) ) ;
#8759=ORIENTED_EDGE ( 'NONE', *, *, #7567, .F. ) ;
#8766=ORIENTED_EDGE ( 'NONE', *, *, #11219, .T. ) ;
#8770=ORIENTED_EDGE ( 'NONE', *, *, #16941, .F. ) ;
#8771=CARTESIAN_POINT ( 'NONE',  ( 99.99999999999987210, -127.0000000000000568, 150.2000000000014381 ) ) ;
#8774=CARTESIAN_POINT ( 'NONE',  ( -280.0000000000000568, 272.9999999999999432, 145.0000000000000284 ) ) ;
#8787=CARTESIAN_POINT ( 'NONE',  ( -281.4928932188135491, -127.0000000000000568, 152.4000000000014268 ) ) ;
#8789=EDGE_CURVE ( 'NONE', #9214, #11652, #13429, .T. ) ;
#8799=CARTESIAN_POINT ( 'NONE',  ( -280.0000000000000000, 270.0000000000000000, -144.9999999999999716 ) ) ;
#8808=DIRECTION ( 'NONE',  ( 0.000000000000000000, -3.495664435217746987E-15, 1.000000000000000000 ) ) ;
#8816=EDGE_CURVE ( 'NONE', #3965, #2180, #23272, .T. ) ;
#8818=CARTESIAN_POINT ( 'NONE',  ( -285.2000000000008981, 30.00000000000101963, -105.0000000000000142 ) ) ;
#8820=FACE_OUTER_BOUND ( 'NONE', #484, .T. ) ;
#8824=VECTOR ( 'NONE', #18976, 1000.000000000000000 ) ;
#8830=EDGE_LOOP ( 'NONE', ( #4777, #15202, #20661, #2331 ) ) ;
#8833=B_SPLINE_SURFACE_WITH_KNOTS ( 'NONE', 1, 3, ( 
 ( #21244, #15587, #14026, #14141, #21471, #6385, #4573, #21822, #14265, #5066 ),
 ( #18424, #18097, #23534, #10882, #12472, #5518, #12934, #9154, #12583, #1550 ),
 ( #1886, #16398, #9039, #23401, #23749, #3474, #16511, #5657, #6859, #5416 ),
 ( #7203, #1657, #8938, #21607, #7340, #19774, #6992, #18311, #14721, #18208 ) ),
 .UNSPECIFIED., .F., .F., .F.,
 ( 2, 1, 1, 2 ),
 ( 4, 2, 2, 2, 4 ),
 ( -0.01000000000000000021, 0.000000000000000000, 1.000000000000000000, 1.010099999999999998 ),
 ( 0.000000000000000000, 0.2500000000000000000, 0.5000000000000000000, 0.7500000000000000000, 1.000000000000000000 ),
 .UNSPECIFIED. ) ;
#8839=EDGE_LOOP ( 'NONE', ( #14071, #8953, #10562, #17132 ) ) ;
#8842=DIRECTION ( 'NONE',  ( 0.000000000000000000, 0.000000000000000000, 1.000000000000000000 ) ) ;
#8845=ADVANCED_FACE ( 'NONE', ( #23740, #8509, #12820 ), #21926, .T. ) ;
#8856=UNCERTAINTY_MEASURE_WITH_UNIT (LENGTH_MEASURE( 1.000000000000000082E-05 ), #11883, 'distance_accuracy_value', 'NONE');
#8860=VECTOR ( 'NONE', #3740, 1000.000000000000000 ) ;
#8862=CARTESIAN_POINT ( 'NONE',  ( 281.4928932188134354, -132.2000000000000455, -150.2000000000013245 ) ) ;
#8864=VECTOR ( 'NONE', #19009, 1000.000000000000000 ) ;
#8865=AXIS2_PLACEMENT_3D ( 'NONE', #18873, #7649, #15160 ) ;
#8881=VECTOR ( 'NONE', #19243, 1000.000000000000000 ) ;
#8888=CARTESIAN_POINT ( 'NONE',  ( -285.2000000000006708, 90.00000000000102318, -32.35000000000004405 ) ) ;
#8894=EDGE_CURVE ( 'NONE', #12339, #539, #21815, .T. ) ;
#8901=DIRECTION ( 'NONE',  ( 0.000000000000000000, -1.000000000000000000, 6.123233995736766036E-17 ) ) ;
#8905=ADVANCED_FACE ( 'NONE', ( #10744 ), #5161, .F. ) ;
#8907=AXIS2_PLACEMENT_3D ( 'NONE', #2136, #2503, #9896 ) ;
#8918=VERTEX_POINT ( 'NONE', #3683 ) ;
#8927=ORIENTED_EDGE ( 'NONE', *, *, #4696, .T. ) ;
#8937=ORIENTED_EDGE ( 'NONE', *, *, #13795, .T. ) ;
#8938=CARTESIAN_POINT ( 'NONE',  ( 280.2488155364687827, 269.9132285165672442, 145.5679143846943475 ) ) ;
#8948=CARTESIAN_POINT ( 'NONE',  ( 285.0646579186752660, 269.1610889986682196, -146.2440776823444537 ) ) ;
#8953=ORIENTED_EDGE ( 'NONE', *, *, #594, .T. ) ;
#8957=LINE ( 'NONE', #21496, #17612 ) ;
#8960=ORIENTED_EDGE ( 'NONE', *, *, #8614, .F. ) ;
#8965=CARTESIAN_POINT ( 'NONE',  ( -281.4928932188134354, 35.00000000000022737, -113.4834095219707848 ) ) ;
#8972=ORIENTED_EDGE ( 'NONE', *, *, #12603, .F. ) ;
#8977=CIRCLE ( 'NONE', #10928, 2.649999999999971934 ) ;
#8978=EDGE_CURVE ( 'NONE', #17822, #21291, #16490, .T. ) ;
#8979=CARTESIAN_POINT ( 'NONE',  ( -285.2000000000014666, -127.0000000000000568, 0.000000000000000000 ) ) ;
#8982=VERTEX_POINT ( 'NONE', #18770 ) ;
#8986=VERTEX_POINT ( 'NONE', #15076 ) ;
#8989=VERTEX_POINT ( 'NONE', #2234 ) ;
#8991=ORIENTED_EDGE ( 'NONE', *, *, #7055, .F. ) ;
#9004=CARTESIAN_POINT ( 'NONE',  ( 280.1255802622536635, 269.9854425596107035, -145.2906609804447555 ) ) ;
#9007=DIRECTION ( 'NONE',  ( -1.000000000000000000, 0.000000000000000000, 0.000000000000000000 ) ) ;
#9008=CARTESIAN_POINT ( 'NONE',  ( 280.7774350431395760, 271.3570580646226631, -148.7968359015655437 ) ) ;
#9010=ORIENTED_EDGE ( 'NONE', *, *, #5550, .T. ) ;
#9016=LINE ( 'NONE', #14361, #1484 ) ;
#9018=ORIENTED_EDGE ( 'NONE', *, *, #11275, .F. ) ;
#9021=DIRECTION ( 'NONE',  ( 0.000000000000000000, -3.495664435217746987E-15, 1.000000000000000000 ) ) ;
#9029=ADVANCED_BREP_SHAPE_REPRESENTATION ( '', ( #12378, #11210 ), #1924 ) ;
#9038=ORIENTED_EDGE ( 'NONE', *, *, #20885, .F. ) ;
#9039=CARTESIAN_POINT ( 'NONE',  ( 280.2488155364687827, 269.9427398886703031, 145.5758453455904373 ) ) ;
#9041=ORIENTED_EDGE ( 'NONE', *, *, #17411, .T. ) ;
#9046=DIRECTION ( 'NONE',  ( -1.000000000000000000, 6.640089860198304064E-16, 0.000000000000000000 ) ) ;
#9050=ORIENTED_EDGE ( 'NONE', *, *, #20562, .T. ) ;
#9051=CARTESIAN_POINT ( 'NONE',  ( 285.2299999999999045, 268.4847249064869743, -146.3684637172358123 ) ) ;
#9064=CIRCLE ( 'NONE', #8294, 5.249999999999949374 ) ;
#9066=CARTESIAN_POINT ( 'NONE',  ( -100.0000000000000853, -127.0000000000000568, 152.4000000000014268 ) ) ;
#9074=LINE ( 'NONE', #5448, #22733 ) ;
#9091=VERTEX_POINT ( 'NONE', #2365 ) ;
#9119=DIRECTION ( 'NONE',  ( -1.000000000000000000, 0.000000000000000000, 0.000000000000000000 ) ) ;
#9122=CARTESIAN_POINT ( 'NONE',  ( 280.4986342070537830, 269.7080393212557397, -146.1045205713627126 ) ) ;
#9124=CARTESIAN_POINT ( 'NONE',  ( -285.2000000000000455, 268.4807971656551331, 146.3684637452624884 ) ) ;
#9131=ORIENTED_EDGE ( 'NONE', *, *, #14512, .T. ) ;
#9135=DIRECTION ( 'NONE',  ( 0.000000000000000000, 0.000000000000000000, 1.000000000000000000 ) ) ;
#9138=LINE ( 'NONE', #16492, #6518 ) ;
#9141=CARTESIAN_POINT ( 'NONE',  ( -282.2000000000012960, -74.99999999999899103, -90.00000000000000000 ) ) ;
#9147=DIRECTION ( 'NONE',  ( 0.000000000000000000, 0.000000000000000000, 1.000000000000000000 ) ) ;
#9152=CARTESIAN_POINT ( 'NONE',  ( -282.2000000000000455, 267.7999999999999545, 145.0000000000000284 ) ) ;
#9154=CARTESIAN_POINT ( 'NONE',  ( 281.2440776823444253, 269.1610889986682196, 150.0646579186752376 ) ) ;
#9170=FACE_OUTER_BOUND ( 'NONE', #3146, .T. ) ;
#9177=EDGE_CURVE ( 'NONE', #16083, #18758, #14213, .T. ) ;
#9180=EDGE_CURVE ( 'NONE', #14990, #23782, #1077, .T. ) ;
#9195=ORIENTED_EDGE ( 'NONE', *, *, #4827, .T. ) ;
#9197=CARTESIAN_POINT ( 'NONE',  ( -285.2000000000014666, -129.2000000000000455, -146.4928932188134070 ) ) ;
#9213=CARTESIAN_POINT ( 'NONE',  ( 280.9952621458755857, 268.9079617568159506, -146.9223300543793016 ) ) ;
#9214=VERTEX_POINT ( 'NONE', #6463 ) ;
#9219=ORIENTED_EDGE ( 'NONE', *, *, #19441, .F. ) ;
#9237=DIRECTION ( 'NONE',  ( 0.000000000000000000, 0.000000000000000000, -1.000000000000000000 ) ) ;
#9249=VERTEX_POINT ( 'NONE', #15902 ) ;
#9258=VERTEX_POINT ( 'NONE', #12185 ) ;
#9259=VECTOR ( 'NONE', #21388, 1000.000000000000000 ) ;
#9274=ORIENTED_EDGE ( 'NONE', *, *, #22005, .F. ) ;
#9280=ORIENTED_EDGE ( 'NONE', *, *, #1972, .F. ) ;
#9281=VECTOR ( 'NONE', #19640, 1000.000000000000000 ) ;
#9297=CARTESIAN_POINT ( 'NONE',  ( -282.2000000000010687, -19.99999999999898392, 105.0000000000000000 ) ) ;
#9299=EDGE_CURVE ( 'NONE', #12117, #16906, #5320, .T. ) ;
#9303=DIRECTION ( 'NONE',  ( 0.000000000000000000, -3.495664435217746987E-15, 1.000000000000000000 ) ) ;
#9306=CARTESIAN_POINT ( 'NONE',  ( -288.2000000000006708, 90.00000000000102318, -32.35000000000004405 ) ) ;
#9324=DIRECTION ( 'NONE',  ( 0.000000000000000000, -1.000000000000000000, 0.000000000000000000 ) ) ;
#9326=CARTESIAN_POINT ( 'NONE',  ( -281.9771650631954572, 268.7755899421579784, -146.0571594757292075 ) ) ;
#9331=ORIENTED_EDGE ( 'NONE', *, *, #13755, .F. ) ;
#9335=ORIENTED_EDGE ( 'NONE', *, *, #13755, .T. ) ;
#9347=ORIENTED_EDGE ( 'NONE', *, *, #16107, .T. ) ;
#9364=CARTESIAN_POINT ( 'NONE',  ( -285.2000000000010687, -19.99999999999898392, 107.6499999999999631 ) ) ;
#9365=CARTESIAN_POINT ( 'NONE',  ( -280.6847249064867924, 273.0299999999999159, -145.1244295015775094 ) ) ;
#9369=CARTESIAN_POINT ( 'NONE',  ( 281.4301685943533471, 268.1431883566702368, -150.1999999999999318 ) ) ;
#9375=CARTESIAN_POINT ( 'NONE',  ( 34.75000000000005684, 100.0000000000000000, 147.2000000000005855 ) ) ;
#9388=CARTESIAN_POINT ( 'NONE',  ( -288.2000000000010687, -19.99999999999898392, 105.0000000000000000 ) ) ;
#9395=EDGE_LOOP ( 'NONE', ( #14433, #20120, #12494, #8750 ) ) ;
#9420=LINE ( 'NONE', #15112, #9484 ) ;
#9421=CARTESIAN_POINT ( 'NONE',  ( 281.4928932188133217, -129.2000000000000455, 152.4000000000014268 ) ) ;
#9425=VERTEX_POINT ( 'NONE', #7645 ) ;
#9432=PLANE ( 'NONE',  #19270 ) ;
#9444=ORIENTED_EDGE ( 'NONE', *, *, #6605, .T. ) ;
#9445=VECTOR ( 'NONE', #6090, 1000.000000000000000 ) ;
#9448=CARTESIAN_POINT ( 'NONE',  ( 280.2488155364688396, 272.8646579186753343, -146.3610889986682366 ) ) ;
#9449=EDGE_CURVE ( 'NONE', #12183, #16906, #289, .T. ) ;
#9459=DIRECTION ( 'NONE',  ( 1.000000000000000000, -3.495664435217746987E-15, -0.000000000000000000 ) ) ;
#9466=CARTESIAN_POINT ( 'NONE',  ( -280.4975000228327531, 272.3132312761073877, 147.6054396500290977 ) ) ;
#9470=PLANE ( 'NONE',  #22904 ) ;
#9471=ORIENTED_EDGE ( 'NONE', *, *, #20927, .F. ) ;
#9472=CARTESIAN_POINT ( 'NONE',  ( -280.9952621458755857, 270.4188186979286570, -149.5436892194421432 ) ) ;
#9473=CARTESIAN_POINT ( 'NONE',  ( 0.000000000000000000, 0.000000000000000000, 0.000000000000000000 ) ) ;
#9479=CARTESIAN_POINT ( 'NONE',  ( 279.9999999999999432, 269.9999999999999432, -144.9999999999999716 ) ) ;
#9484=VECTOR ( 'NONE', #18572, 1000.000000000000000 ) ;
#9488=CARTESIAN_POINT ( 'NONE',  ( -280.0000000000000568, 272.9999999999999432, -144.9999999999999716 ) ) ;
#9489=ORIENTED_EDGE ( 'NONE', *, *, #15221, .T. ) ;
#9504=ORIENTED_EDGE ( 'NONE', *, *, #12038, .T. ) ;
#9505=EDGE_CURVE ( 'NONE', #10284, #10987, #4628, .T. ) ;
#9507=CARTESIAN_POINT ( 'NONE',  ( 40.00000000000000000, 100.0000000000000000, 150.2000000000009550 ) ) ;
#9514=EDGE_CURVE ( 'NONE', #14837, #10284, #16832, .T. ) ;
#9520=ADVANCED_FACE ( 'NONE', ( #2200 ), #15158, .T. ) ;
#9523=CARTESIAN_POINT ( 'NONE',  ( -312.2000000000014666, -129.2000000000000455, 146.4928932188134638 ) ) ;
#9524=VERTEX_POINT ( 'NONE', #3038 ) ;
#9525=CARTESIAN_POINT ( 'NONE',  ( 280.2880230824752061, 269.9999999999999432, -145.1244266708878001 ) ) ;
#9533=DIRECTION ( 'NONE',  ( -1.000000000000000000, 0.000000000000000000, -0.000000000000000000 ) ) ;
#9534=PRODUCT_DEFINITION_CONTEXT ( 'detailed design', #20316, 'design' ) ;
#9545=EDGE_LOOP ( 'NONE', ( #21331, #11457, #1203, #21195 ) ) ;
#9548=DIRECTION ( 'NONE',  ( -1.000000000000000000, -0.000000000000000000, -0.000000000000000000 ) ) ;
#9550=CARTESIAN_POINT ( 'NONE',  ( -282.2000000000006708, 90.00000000000100897, 34.99999999999999289 ) ) ;
#9552=CARTESIAN_POINT ( 'NONE',  ( -45.00000000000000000, 272.9999999999999432, 5.249999999999973355 ) ) ;
#9562=ORIENTED_EDGE ( 'NONE', *, *, #7960, .F. ) ;
#9564=CARTESIAN_POINT ( 'NONE',  ( 280.4976310729377929, 272.3699028110927998, -147.6339272673397716 ) ) ;
#9573=DIRECTION ( 'NONE',  ( -1.000000000000000000, 3.495664435217746592E-15, -0.000000000000000000 ) ) ;
#9589=CARTESIAN_POINT ( 'NONE',  ( -280.0000000000000000, 270.0000000000000000, -144.9999999999999716 ) ) ;
#9594=CARTESIAN_POINT ( 'NONE',  ( 34.75000000000005684, 100.0000000000000000, 150.2000000000009550 ) ) ;
#9613=VECTOR ( 'NONE', #14348, 1000.000000000000000 ) ;
#9617=ORIENTED_EDGE ( 'NONE', *, *, #515, .F. ) ;
#9620=VECTOR ( 'NONE', #22818, 1000.000000000000000 ) ;
#9631=VECTOR ( 'NONE', #20791, 1000.000000000000000 ) ;
#9635=ADVANCED_FACE ( 'NONE', ( #8501 ), #15875, .T. ) ;
#9636=ORIENTED_EDGE ( 'NONE', *, *, #12122, .T. ) ;
#9645=CARTESIAN_POINT ( 'NONE',  ( 281.6574776399288567, 269.2538215477169956, -145.8086578304521197 ) ) ;
#9656=CARTESIAN_POINT ( 'NONE',  ( -100.0000000000000853, -127.0000000000000568, 150.2000000000014381 ) ) ;
#9659=FACE_OUTER_BOUND ( 'NONE', #23335, .T. ) ;
#9675=DIRECTION ( 'NONE',  ( -0.000000000000000000, -1.000000000000000000, 6.123233995736766036E-17 ) ) ;
#9676=PRODUCT_DEFINITION_FORMATION_WITH_SPECIFIED_SOURCE ( 'ANY', '', #4766, .NOT_KNOWN. ) ;
#9685=EDGE_LOOP ( 'NONE', ( #21298, #18941, #22264, #5896 ) ) ;
#9688=DIRECTION ( 'NONE',  ( -0.000000000000000000, 6.982962677686266711E-15, -1.000000000000000000 ) ) ;
#9689=CARTESIAN_POINT ( 'NONE',  ( -281.9094021484634709, 268.9021437883071712, -145.9954397628183926 ) ) ;
#9692=DIRECTION ( 'NONE',  ( 1.000000000000000000, -0.000000000000000000, 0.000000000000000000 ) ) ;
#9699=CARTESIAN_POINT ( 'NONE',  ( 280.2488155364688396, 269.9427398886703600, -145.5758453455903805 ) ) ;
#9702=ORIENTED_EDGE ( 'NONE', *, *, #17314, .T. ) ;
#9706=ORIENTED_EDGE ( 'NONE', *, *, #6154, .F. ) ;
#9710=DIRECTION ( 'NONE',  ( -3.495664435217746987E-15, 1.000000000000000000, 0.000000000000000000 ) ) ;
#9716=CARTESIAN_POINT ( 'NONE',  ( -281.7484459290826635, 269.1429506979391704, 145.8703180930665440 ) ) ;
#9724=CARTESIAN_POINT ( 'NONE',  ( 281.3520027839447835, 269.5592670532759030, 145.6220388411722695 ) ) ;
#9725=CARTESIAN_POINT ( 'NONE',  ( -280.0000000000000568, 269.9999999999999432, 145.0000000000000284 ) ) ;
#9728=LINE ( 'NONE', #11683, #16476 ) ;
#9738=CARTESIAN_POINT ( 'NONE',  ( -288.2000000000010687, -19.99999999999898392, 105.0000000000000000 ) ) ;
#9750=DIRECTION ( 'NONE',  ( 0.000000000000000000, 0.000000000000000000, 1.000000000000000000 ) ) ;
#9765=CARTESIAN_POINT ( 'NONE',  ( 279.9999999999999432, 267.7999999999999545, 146.4928932188134922 ) ) ;
#9768=DIRECTION ( 'NONE',  ( -1.000000000000000000, -0.000000000000000000, -0.000000000000000000 ) ) ;
#9771=SHAPE_REPRESENTATION ( 'head cover', ( #11210 ), #1924 ) ;
#9777=EDGE_LOOP ( 'NONE', ( #16817, #10659, #14772, #13700 ) ) ;
#9780=AXIS2_PLACEMENT_3D ( 'NONE', #1226, #6901, #14304 ) ;
#9786=EDGE_CURVE ( 'NONE', #13791, #10471, #1162, .T. ) ;
#9798=CIRCLE ( 'NONE', #10967, 5.249999999999973355 ) ;
#9800=CARTESIAN_POINT ( 'NONE',  ( 283.7968359015656006, 271.3570580646228336, 145.7774350431395760 ) ) ;
#9803=CARTESIAN_POINT ( 'NONE',  ( -312.2000000000014666, -132.2000000000000455, 146.4928932188134638 ) ) ;
#9805=PLANE ( 'NONE',  #23795 ) ;
#9824=VERTEX_POINT ( 'NONE', #22465 ) ;
#9825=EDGE_CURVE ( 'NONE', #22918, #12463, #4104, .T. ) ;
#9828=DIRECTION ( 'NONE',  ( 0.000000000000000000, 1.000000000000000000, -4.183096374613631247E-18 ) ) ;
#9830=LINE ( 'NONE', #2998, #8824 ) ;
#9833=DIRECTION ( 'NONE',  ( 0.000000000000000000, 0.000000000000000000, 1.000000000000000000 ) ) ;
#9835=CARTESIAN_POINT ( 'NONE',  ( -280.1244294735509470, 273.0000000000000000, -145.6807971656549796 ) ) ;
#9838=VECTOR ( 'NONE', #4780, 1000.000000000000000 ) ;
#9842=CARTESIAN_POINT ( 'NONE',  ( 285.2299999999999045, 267.7999999999999545, 146.4928932188134922 ) ) ;
#9848=CARTESIAN_POINT ( 'NONE',  ( 287.4000000000013415, -127.0000000000000568, -146.4928932188134070 ) ) ;
#9851=ORIENTED_EDGE ( 'NONE', *, *, #23412, .T. ) ;
#9853=CARTESIAN_POINT ( 'NONE',  ( -281.4928932188135491, -132.2000000000000455, 152.4000000000014268 ) ) ;
#9856=DIRECTION ( 'NONE',  ( 3.495664435217746592E-15, 1.000000000000000000, 7.709882115452476934E-17 ) ) ;
#9857=DIRECTION ( 'NONE',  ( 1.000000000000000000, 0.000000000000000000, 0.000000000000000000 ) ) ;
#9861=CARTESIAN_POINT ( 'NONE',  ( 0.000000000000000000, 0.000000000000000000, -177.2000000000013529 ) ) ;
#9865=CARTESIAN_POINT ( 'NONE',  ( -282.2000000000011255, -29.99999999999898037, -102.3500000000000227 ) ) ;
#9866=AXIS2_PLACEMENT_3D ( 'NONE', #7725, #6018, #17259 ) ;
#9876=CARTESIAN_POINT ( 'NONE',  ( -288.2000000000008981, 30.00000000000101963, -107.6499999999999773 ) ) ;
#9887=CARTESIAN_POINT ( 'NONE',  ( 280.2489140339769165, 272.8335297745771300, 146.3488036478619563 ) ) ;
#9894=CIRCLE ( 'NONE', #17962, 5.249999999999991118 ) ;
#9896=DIRECTION ( 'NONE',  ( -3.495664435217746987E-15, -1.000000000000000000, 0.000000000000000000 ) ) ;
#9899=CARTESIAN_POINT ( 'NONE',  ( 0.000000000000000000, 0.000000000000000000, -150.2000000000008981 ) ) ;
#9903=ORIENTED_EDGE ( 'NONE', *, *, #8579, .F. ) ;
#9905=DIRECTION ( 'NONE',  ( 0.000000000000000000, 0.000000000000000000, -1.000000000000000000 ) ) ;
#9907=ORIENTED_EDGE ( 'NONE', *, *, #23141, .T. ) ;
#9912=ORIENTED_EDGE ( 'NONE', *, *, #6359, .F. ) ;
#9913=VECTOR ( 'NONE', #263, 1000.000000000000000 ) ;
#9933=AXIS2_PLACEMENT_3D ( 'NONE', #6024, #22441, #16778 ) ;
#9942=CARTESIAN_POINT ( 'NONE',  ( -281.4928932188135491, 267.7999999999999545, 150.2299999999999898 ) ) ;
#9945=ORIENTED_EDGE ( 'NONE', *, *, #20772, .F. ) ;
#9951=PLANE ( 'NONE',  #23453 ) ;
#9981=DIRECTION ( 'NONE',  ( 1.000000000000000000, 0.000000000000000000, 0.000000000000000000 ) ) ;
#9988=CARTESIAN_POINT ( 'NONE',  ( -287.4000000000014552, -127.0000000000000568, 146.4928932188134638 ) ) ;
#9989=AXIS2_PLACEMENT_3D ( 'NONE', #6876, #10535, #5188 ) ;
#9997=PLANE ( 'NONE',  #1925 ) ;
#10006=LINE ( 'NONE', #19027, #851 ) ;
#10007=AXIS2_PLACEMENT_3D ( 'NONE', #9899, #17380, #822 ) ;
#10021=UNCERTAINTY_MEASURE_WITH_UNIT (LENGTH_MEASURE( 1.000000000000000082E-05 ), #21885, 'distance_accuracy_value', 'NONE');
#10053=VECTOR ( 'NONE', #7022, 1000.000000000000000 ) ;
#10055=CARTESIAN_POINT ( 'NONE',  ( 45.24999999999994316, 100.0000000000000000, 150.2000000000009550 ) ) ;
#10060=( NAMED_UNIT ( * ) SI_UNIT ( $, .STERADIAN. ) SOLID_ANGLE_UNIT ( ) );
#10068=B_SPLINE_CURVE_WITH_KNOTS ( 'NONE', 3,
 ( #13188, #16757, #18921, #9887, #6255, #15453, #15093, #2380, #17243, #20866, #22657, #22423, #6129, #13295, #5883, #18786, #4318, #22791, #13661, #2251 ),
 .UNSPECIFIED., .F., .F.,
 ( 4, 2, 2, 2, 2, 2, 2, 2, 2, 4 ),
 ( 0.000000000000000000, 0.001035985217005689577, 0.002071970434011379154, 0.003107955651017068298, 0.003625948259519924579, 0.004143940868022780860, 0.005179926085028581026, 0.006215911302034382926, 0.007251896519040183092, 0.008287881736045983258 ),
 .UNSPECIFIED. ) ;
#10069=DIRECTION ( 'NONE',  ( 1.000000000000000000, 0.000000000000000000, 0.000000000000000000 ) ) ;
#10070=EDGE_LOOP ( 'NONE', ( #15198, #9903, #10821, #19955 ) ) ;
#10081=EDGE_CURVE ( 'NONE', #18466, #21466, #16641, .T. ) ;
#10100=CARTESIAN_POINT ( 'NONE',  ( -280.0000000000000568, 267.7999999999999545, -146.4928932188134354 ) ) ;
#10109=LINE ( 'NONE', #18890, #21377 ) ;
#10112=CARTESIAN_POINT ( 'NONE',  ( 279.9999999999999432, 267.7999999999999545, 147.1999999999999886 ) ) ;
#10122=LINE ( 'NONE', #19615, #1115 ) ;
#10135=CARTESIAN_POINT ( 'NONE',  ( 279.9999999999999432, 272.9999999999999432, 145.0000000000000284 ) ) ;
#10137=ADVANCED_FACE ( 'NONE', ( #14834 ), #7199, .T. ) ;
#10149=ORIENTED_EDGE ( 'NONE', *, *, #4891, .F. ) ;
#10151=EDGE_CURVE ( 'NONE', #15299, #2147, #21932, .T. ) ;
#10154=EDGE_CURVE ( 'NONE', #5006, #21142, #7337, .T. ) ;
#10180=ADVANCED_FACE ( 'NONE', ( #22165 ), #3687, .T. ) ;
#10181=CARTESIAN_POINT ( 'NONE',  ( 281.4928932188133786, -127.0000000000000568, 150.2000000000013813 ) ) ;
#10183=DIRECTION ( 'NONE',  ( 0.000000000000000000, 0.000000000000000000, 1.000000000000000000 ) ) ;
#10193=ORIENTED_EDGE ( 'NONE', *, *, #20975, .F. ) ;
#10197=FACE_OUTER_BOUND ( 'NONE', #5675, .T. ) ;
#10199=CARTESIAN_POINT ( 'NONE',  ( -285.2000000000000455, 267.7999999999999545, -146.4928932188134354 ) ) ;
#10234=ADVANCED_FACE ( 'NONE', ( #13762 ), #9997, .F. ) ;
#10255=CARTESIAN_POINT ( 'NONE',  ( -283.5570580646227086, 271.5968359015654983, 145.7154581756739162 ) ) ;
#10280=FACE_OUTER_BOUND ( 'NONE', #10782, .T. ) ;
#10281=AXIS2_PLACEMENT_3D ( 'NONE', #7171, #12547, #3656 ) ;
#10284=VERTEX_POINT ( 'NONE', #13283 ) ;
#10288=ORIENTED_EDGE ( 'NONE', *, *, #6927, .F. ) ;
#10300=CARTESIAN_POINT ( 'NONE',  ( 281.4928932188133217, -132.2000000000000455, 152.4000000000014268 ) ) ;
#10304=DIRECTION ( 'NONE',  ( -0.000000000000000000, -0.000000000000000000, 1.000000000000000000 ) ) ;
#10306=CARTESIAN_POINT ( 'NONE',  ( 282.2000000000013529, -127.0000000000000568, 146.4928932188134638 ) ) ;
#10313=DIRECTION ( 'NONE',  ( 1.000000000000000000, 0.000000000000000000, 0.000000000000000000 ) ) ;
#10316=CARTESIAN_POINT ( 'NONE',  ( -282.1427398886704054, 268.3758453455903918, -146.2440776823445390 ) ) ;
#10326=EDGE_CURVE ( 'NONE', #14070, #21880, #16133, .T. ) ;
#10327=VECTOR ( 'NONE', #4233, 1000.000000000000000 ) ;
#10331=ORIENTED_EDGE ( 'NONE', *, *, #20806, .F. ) ;
#10352=DIRECTION ( 'NONE',  ( -0.000000000000000000, -0.000000000000000000, 1.000000000000000000 ) ) ;
#10357=CARTESIAN_POINT ( 'NONE',  ( -284.5135885331259260, 270.4045710003934460, -145.9955614683502176 ) ) ;
#10374=PLANE ( 'NONE',  #23547 ) ;
#10382=CARTESIAN_POINT ( 'NONE',  ( -280.8703180930666576, 269.1429506979392272, -146.7484459290826067 ) ) ;
#10387=LINE ( 'NONE', #8121, #3760 ) ;
#10393=CARTESIAN_POINT ( 'NONE',  ( 281.4928932188133217, -127.0000000000000568, 147.2000000000014381 ) ) ;
#10396=AXIS2_PLACEMENT_3D ( 'NONE', #18215, #14169, #3830 ) ;
#10397=ORIENTED_EDGE ( 'NONE', *, *, #14082, .T. ) ;
#10406=EDGE_CURVE ( 'NONE', #15945, #16256, #11954, .T. ) ;
#10412=AXIS2_PLACEMENT_3D ( 'NONE', #16124, #10592, #16010 ) ;
#10435=DIRECTION ( 'NONE',  ( -1.000000000000000000, 3.495664435217746987E-15, 0.000000000000000000 ) ) ;
#10438=FACE_OUTER_BOUND ( 'NONE', #14977, .T. ) ;
#10441=EDGE_CURVE ( 'NONE', #15992, #14150, #10122, .T. ) ;
#10447=AXIS2_PLACEMENT_3D ( 'NONE', #6678, #21398, #3393 ) ;
#10458=ORIENTED_EDGE ( 'NONE', *, *, #6359, .T. ) ;
#10461=CARTESIAN_POINT ( 'NONE',  ( 282.2000000000013529, -127.0000000000000568, 145.0000000000000284 ) ) ;
#10467=DIRECTION ( 'NONE',  ( 0.000000000000000000, 0.000000000000000000, 1.000000000000000000 ) ) ;
#10471=VERTEX_POINT ( 'NONE', #8771 ) ;
#10472=( NAMED_UNIT ( * ) PLANE_ANGLE_UNIT ( ) SI_UNIT ( $, .RADIAN. ) );
#10482=DIRECTION ( 'NONE',  ( 1.000000000000000000, 0.000000000000000000, 0.000000000000000000 ) ) ;
#10490=CARTESIAN_POINT ( 'NONE',  ( -280.0000000000000568, 269.9696999999999889, 145.0000000000000284 ) ) ;
#10502=FACE_OUTER_BOUND ( 'NONE', #14811, .T. ) ;
#10509=CARTESIAN_POINT ( 'NONE',  ( -284.9324007871372828, 269.4810649015074659, 146.1807969192697954 ) ) ;
#10511=ORIENTED_EDGE ( 'NONE', *, *, #23275, .T. ) ;
#10512=DIRECTION ( 'NONE',  ( -1.000000000000000000, -0.000000000000000000, -0.000000000000000000 ) ) ;
#10516=EDGE_CURVE ( 'NONE', #19505, #15324, #2958, .T. ) ;
#10534=CARTESIAN_POINT ( 'NONE',  ( -280.6845057130643681, 271.7107452280324082, -148.4314821058792404 ) ) ;
#10535=DIRECTION ( 'NONE',  ( 1.000000000000000000, -3.495664435217746987E-15, -0.000000000000000000 ) ) ;
#10537=ORIENTED_EDGE ( 'NONE', *, *, #20858, .F. ) ;
#10542=ADVANCED_FACE ( 'NONE', ( #16474 ), #10848, .F. ) ;
#10546=EDGE_CURVE ( 'NONE', #1647, #22518, #17730, .T. ) ;
#10548=DIRECTION ( 'NONE',  ( -1.000000000000000000, 0.000000000000000000, 0.000000000000000000 ) ) ;
#10549=EDGE_CURVE ( 'NONE', #2171, #23104, #19626, .T. ) ;
#10559=VERTEX_POINT ( 'NONE', #10957 ) ;
#10561=ORIENTED_EDGE ( 'NONE', *, *, #12377, .F. ) ;
#10562=ORIENTED_EDGE ( 'NONE', *, *, #18293, .T. ) ;
#10583=ORIENTED_EDGE ( 'NONE', *, *, #18003, .T. ) ;
#10592=DIRECTION ( 'NONE',  ( -1.000000000000000000, -0.000000000000000000, -0.000000000000000000 ) ) ;
#10594=VERTEX_POINT ( 'NONE', #9364 ) ;
#10599=DIRECTION ( 'NONE',  ( -1.000000000000000000, -0.000000000000000000, -0.000000000000000000 ) ) ;
#10604=AXIS2_PLACEMENT_3D ( 'NONE', #18859, #13248, #18731 ) ;
#10605=DIRECTION ( 'NONE',  ( -0.000000000000000000, -0.000000000000000000, -1.000000000000000000 ) ) ;
#10606=CARTESIAN_POINT ( 'NONE',  ( -284.6730547946947354, 270.1059783239178387, -146.0571358042175802 ) ) ;
#10619=AXIS2_PLACEMENT_3D ( 'NONE', #17668, #15754, #1128 ) ;
#10626=DIRECTION ( 'NONE',  ( 0.000000000000000000, -1.000000000000000000, 0.000000000000000000 ) ) ;
#10632=ORIENTED_EDGE ( 'NONE', *, *, #8978, .F. ) ;
#10634=EDGE_CURVE ( 'NONE', #15403, #16905, #18059, .T. ) ;
#10636=EDGE_LOOP ( 'NONE', ( #9331, #11990 ) ) ;
#10643=ADVANCED_FACE ( 'NONE', ( #4277 ), #13144, .T. ) ;
#10644=ADVANCED_FACE ( 'NONE', ( #20818 ), #18268, .F. ) ;
#10646=ORIENTED_EDGE ( 'NONE', *, *, #1075, .F. ) ;
#10659=ORIENTED_EDGE ( 'NONE', *, *, #2643, .T. ) ;
#10660=PLANE ( 'NONE',  #12554 ) ;
#10673=CARTESIAN_POINT ( 'NONE',  ( -280.6225751257470620, 269.5484459290826180, 146.3429506979392443 ) ) ;
#10679=DIRECTION ( 'NONE',  ( -0.000000000000000000, -0.000000000000000000, 1.000000000000000000 ) ) ;
#10685=VERTEX_POINT ( 'NONE', #10199 ) ;
#10693=CARTESIAN_POINT ( 'NONE',  ( -287.4000000000014552, -127.0000000000000568, -146.4928932188134070 ) ) ;
#10701=CARTESIAN_POINT ( 'NONE',  ( -282.2000000000000455, 267.7999999999999545, 146.4928932188134354 ) ) ;
#10721=CARTESIAN_POINT ( 'NONE',  ( -282.6188186979287025, 272.3436892194421262, 145.4976310729378213 ) ) ;
#10723=CARTESIAN_POINT ( 'NONE',  ( -288.2000000000013529, -89.99999999999897682, 24.33333333333333215 ) ) ;
#10734=LINE ( 'NONE', #23732, #11192 ) ;
#10744=FACE_OUTER_BOUND ( 'NONE', #18924, .T. ) ;
#10746=EDGE_LOOP ( 'NONE', ( #9335, #3901, #9347, #19071 ) ) ;
#10764=CARTESIAN_POINT ( 'NONE',  ( 280.6847249064868492, 273.0299999999999159, -145.1244295015775378 ) ) ;
#10775=EDGE_CURVE ( 'NONE', #21417, #16062, #17659, .T. ) ;
#10779=CIRCLE ( 'NONE', #341, 2.649999999999975486 ) ;
#10782=EDGE_LOOP ( 'NONE', ( #2830, #3469, #3754, #16703 ) ) ;
#10785=B_SPLINE_SURFACE_WITH_KNOTS ( 'NONE', 1, 3, ( 
 ( #14320, #4106, #15250, #2308, #2175, #13463, #9564, #5694, #5932, #11519 ),
 ( #22354, #16578, #15136, #16927, #22466, #7758, #396, #9448, #3748, #13228 ),
 ( #16692, #11164, #5574, #9213, #18493, #20776, #4240, #9699, #13340, #22584 ),
 ( #12985, #6047, #17053, #18365, #14770, #22103, #44, #7500, #1820, #7389 ) ),
 .UNSPECIFIED., .F., .F., .F.,
 ( 2, 1, 1, 2 ),
 ( 4, 2, 2, 2, 4 ),
 ( -0.01000000000000000021, 0.000000000000000000, 1.000000000000000000, 1.010099999999999998 ),
 ( 0.000000000000000000, 0.2500000000000000000, 0.5000000000000000000, 0.7500000000000000000, 1.000000000000000000 ),
 .UNSPECIFIED. ) ;
#10791=ORIENTED_EDGE ( 'NONE', *, *, #11069, .F. ) ;
#10793=DIRECTION ( 'NONE',  ( 1.000000000000000000, -0.000000000000000000, -0.000000000000000000 ) ) ;
#10796=CARTESIAN_POINT ( 'NONE',  ( -288.2000000000013529, -89.99999999999896261, -40.33333333333332860 ) ) ;
#10800=CARTESIAN_POINT ( 'NONE',  ( -288.2000000000006708, 90.00000000000100897, 34.99999999999999289 ) ) ;
#10809=CYLINDRICAL_SURFACE ( 'NONE', #14224, 2.649999999999971934 ) ;
#10812=AXIS2_PLACEMENT_3D ( 'NONE', #6705, #21426, #17815 ) ;
#10821=ORIENTED_EDGE ( 'NONE', *, *, #5335, .T. ) ;
#10824=EDGE_CURVE ( 'NONE', #12957, #18256, #8091, .T. ) ;
#10840=CYLINDRICAL_SURFACE ( 'NONE', #11984, 2.199999999999979750 ) ;
#10848=PLANE ( 'NONE',  #19251 ) ;
#10858=CARTESIAN_POINT ( 'NONE',  ( 280.9020829022173302, 270.8299054689547347, -149.2295083325147687 ) ) ;
#10859=EDGE_LOOP ( 'NONE', ( #10331, #2352 ) ) ;
#10861=EDGE_LOOP ( 'NONE', ( #18936, #6711 ) ) ;
#10870=DIRECTION ( 'NONE',  ( -1.000000000000000000, -0.000000000000000000, -0.000000000000000000 ) ) ;
#10882=CARTESIAN_POINT ( 'NONE',  ( 280.4976310729377360, 272.3436892194421262, 147.6188186979287025 ) ) ;
#10913=LINE ( 'NONE', #9197, #3067 ) ;
#10915=ADVANCED_FACE ( 'NONE', ( #15601 ), #20896, .F. ) ;
#10922=ORIENTED_EDGE ( 'NONE', *, *, #12689, .F. ) ;
#10928=AXIS2_PLACEMENT_3D ( 'NONE', #9297, #23757, #14603 ) ;
#10936=VERTEX_POINT ( 'NONE', #5389 ) ;
#10937=AXIS2_PLACEMENT_3D ( 'NONE', #14286, #21488, #6403 ) ;
#10940=ORIENTED_EDGE ( 'NONE', *, *, #5772, .F. ) ;
#10944=CARTESIAN_POINT ( 'NONE',  ( -285.2000000000011255, -29.99999999999898037, -105.0000000000000000 ) ) ;
#10949=EDGE_LOOP ( 'NONE', ( #7844, #813, #13042, #3493 ) ) ;
#10953=LINE ( 'NONE', #18275, #3089 ) ;
#10957=CARTESIAN_POINT ( 'NONE',  ( 281.4928932188133786, -127.0000000000000568, 150.2000000000013813 ) ) ;
#10961=CARTESIAN_POINT ( 'NONE',  ( 280.2494876630255476, 272.8327955282143193, -146.3518577254344564 ) ) ;
#10965=EDGE_LOOP ( 'NONE', ( #19461, #22408, #21655, #12171 ) ) ;
#10967=AXIS2_PLACEMENT_3D ( 'NONE', #15266, #2792, #10183 ) ;
#10984=CARTESIAN_POINT ( 'NONE',  ( -45.00000000000000000, 272.9999999999999432, 0.000000000000000000 ) ) ;
#10987=VERTEX_POINT ( 'NONE', #12907 ) ;
#10989=CARTESIAN_POINT ( 'NONE',  ( 0.000000000000000000, -132.2000000000000455, -177.2000000000013529 ) ) ;
#10995=EDGE_LOOP ( 'NONE', ( #12555, #17572, #8960, #5945 ) ) ;
#10998=CARTESIAN_POINT ( 'NONE',  ( -281.4928932188135491, -132.2000000000000455, 177.2000000000014097 ) ) ;
#10999=ORIENTED_EDGE ( 'NONE', *, *, #6154, .T. ) ;
#11012=CIRCLE ( 'NONE', #19066, 2.649999999999971934 ) ;
#11020=ORIENTED_EDGE ( 'NONE', *, *, #17842, .T. ) ;
#11024=ORIENTED_EDGE ( 'NONE', *, *, #6803, .T. ) ;
#11038=ORIENTED_EDGE ( 'NONE', *, *, #18749, .T. ) ;
#11040=AXIS2_PLACEMENT_3D ( 'NONE', #23166, #13681, #15934 ) ;
#11045=CARTESIAN_POINT ( 'NONE',  ( -40.00000000000000000, 100.0000000000000000, 150.2000000000009550 ) ) ;
#11053=ORIENTED_EDGE ( 'NONE', *, *, #2615, .T. ) ;
#11054=AXIS2_PLACEMENT_3D ( 'NONE', #662, #22763, #2719 ) ;
#11064=EDGE_LOOP ( 'NONE', ( #15448, #5119 ) ) ;
#11069=EDGE_CURVE ( 'NONE', #2779, #10987, #4651, .T. ) ;
#11072=CARTESIAN_POINT ( 'NONE',  ( 281.0571594757293497, 268.7755899421583763, -146.9771650631952582 ) ) ;
#11078=CARTESIAN_POINT ( 'NONE',  ( 0.000000000000000000, 5.068713431065764784E-13, -147.2000000000008981 ) ) ;
#11106=EDGE_CURVE ( 'NONE', #13119, #8023, #2868, .T. ) ;
#11123=DIRECTION ( 'NONE',  ( 0.000000000000000000, -1.000000000000000000, 0.000000000000000000 ) ) ;
#11134=DIRECTION ( 'NONE',  ( -1.000000000000000000, -9.912705577010325549E-17, -3.465149234233960866E-31 ) ) ;
#11141=EDGE_CURVE ( 'NONE', #13958, #17412, #13628, .T. ) ;
#11153=CARTESIAN_POINT ( 'NONE',  ( -280.9755403010747159, 269.7771302778487552, -145.4357197208657055 ) ) ;
#11156=DIRECTION ( 'NONE',  ( 0.000000000000000000, -0.000000000000000000, 1.000000000000000000 ) ) ;
#11164=CARTESIAN_POINT ( 'NONE',  ( 281.3684665479255500, 268.0880230824753312, -147.1999999999999318 ) ) ;
#11169=CIRCLE ( 'NONE', #2245, 2.649999999999971934 ) ;
#11172=CIRCLE ( 'NONE', #7669, 2.649999999999971934 ) ;
#11176=EDGE_CURVE ( 'NONE', #22022, #12343, #13857, .T. ) ;
#11192=VECTOR ( 'NONE', #14367, 1000.000000000000000 ) ;
#11196=AXIS2_PLACEMENT_3D ( 'NONE', #11880, #19189, #11509 ) ;
#11205=DIRECTION ( 'NONE',  ( 0.000000000000000000, -1.000000000000000000, 0.000000000000000000 ) ) ;
#11209=CARTESIAN_POINT ( 'NONE',  ( -282.2000000000011255, -29.99999999999898037, -107.6499999999999631 ) ) ;
#11210=AXIS2_PLACEMENT_3D ( 'NONE', #9473, #14914, #3769 ) ;
#11217=DIRECTION ( 'NONE',  ( -1.000000000000000000, -0.000000000000000000, -0.000000000000000000 ) ) ;
#11219=EDGE_CURVE ( 'NONE', #12822, #7386, #9064, .T. ) ;
#11221=FACE_OUTER_BOUND ( 'NONE', #14222, .T. ) ;
#11234=AXIS2_PLACEMENT_3D ( 'NONE', #16507, #5282, #13047 ) ;
#11240=EDGE_LOOP ( 'NONE', ( #2641, #22906, #22110, #1767 ) ) ;
#11241=CARTESIAN_POINT ( 'NONE',  ( -285.2000000000000455, 269.9999999999999432, -146.4928932188134070 ) ) ;
#11247=CARTESIAN_POINT ( 'NONE',  ( -285.2000000000011255, -29.99999999999898037, -105.0000000000000000 ) ) ;
#11254=FACE_BOUND ( 'NONE', #5305, .T. ) ;
#11265=DIRECTION ( 'NONE',  ( -1.000000000000000000, -0.000000000000000000, -0.000000000000000000 ) ) ;
#11266=CARTESIAN_POINT ( 'NONE',  ( 281.4928932188134354, -127.0000000000000568, -152.4000000000012847 ) ) ;
#11267=ORIENTED_EDGE ( 'NONE', *, *, #22085, .T. ) ;
#11271=CARTESIAN_POINT ( 'NONE',  ( 281.4928932188134354, -129.2000000000000455, -177.2000000000013529 ) ) ;
#11274=DIRECTION ( 'NONE',  ( 1.000000000000000000, -3.495664435217746987E-15, -0.000000000000000000 ) ) ;
#11275=EDGE_CURVE ( 'NONE', #8989, #4643, #14472, .T. ) ;
#11277=EDGE_CURVE ( 'NONE', #2262, #20612, #4755, .T. ) ;
#11281=VERTEX_POINT ( 'NONE', #14085 ) ;
#11283=LINE ( 'NONE', #6041, #10327 ) ;
#11288=EDGE_CURVE ( 'NONE', #13791, #12343, #12285, .T. ) ;
#11293=VERTEX_POINT ( 'NONE', #14201 ) ;
#11299=CARTESIAN_POINT ( 'NONE',  ( 99.99999999999997158, 34.99999999999995026, 147.2000000000010971 ) ) ;
#11309=CARTESIAN_POINT ( 'NONE',  ( -281.4533442688713762, 269.4578961534456312, 145.6839617489740988 ) ) ;
#11316=EDGE_CURVE ( 'NONE', #9249, #2180, #13440, .T. ) ;
#11327=CARTESIAN_POINT ( 'NONE',  ( -280.0000000000000568, 272.9999999999999432, 145.0000000000000284 ) ) ;
#11343=LINE ( 'NONE', #9876, #17666 ) ;
#11347=DIRECTION ( 'NONE',  ( 0.000000000000000000, 0.000000000000000000, 1.000000000000000000 ) ) ;
#11352=DIRECTION ( 'NONE',  ( 0.000000000000000000, -0.000000000000000000, 1.000000000000000000 ) ) ;
#11365=LINE ( 'NONE', #22435, #4454 ) ;
#11366=EDGE_CURVE ( 'NONE', #12940, #9524, #14992, .T. ) ;
#11376=ORIENTED_EDGE ( 'NONE', *, *, #19779, .T. ) ;
#11384=CARTESIAN_POINT ( 'NONE',  ( -280.1245861693740267, 272.9663417894422537, -145.6816199723480452 ) ) ;
#11392=DIRECTION ( 'NONE',  ( 0.000000000000000000, 0.000000000000000000, 1.000000000000000000 ) ) ;
#11394=EDGE_LOOP ( 'NONE', ( #8991, #16420, #17074, #15796 ) ) ;
#11406=ORIENTED_EDGE ( 'NONE', *, *, #62, .T. ) ;
#11424=CARTESIAN_POINT ( 'NONE',  ( -280.2488155364688964, 269.9132285165672442, -145.5679143846942907 ) ) ;
#11428=CARTESIAN_POINT ( 'NONE',  ( -281.4928932188134922, -127.0000000000000568, 150.2000000000013813 ) ) ;
#11430=CARTESIAN_POINT ( 'NONE',  ( 281.3333820183295302, 269.5350371479512432, 145.6220388411722695 ) ) ;
#11432=CIRCLE ( 'NONE', #11054, 2.649999999999971934 ) ;
#11442=AXIS2_PLACEMENT_3D ( 'NONE', #16144, #3667, #12559 ) ;
#11444=CARTESIAN_POINT ( 'NONE',  ( -285.2000000000008981, 35.00000000000100897, 105.0000000000000000 ) ) ;
#11449=CARTESIAN_POINT ( 'NONE',  ( -40.00000000000000000, 100.0000000000000000, -147.2000000000005571 ) ) ;
#11457=ORIENTED_EDGE ( 'NONE', *, *, #19119, .F. ) ;
#11459=CARTESIAN_POINT ( 'NONE',  ( 281.4928932188133217, -127.0000000000000568, 152.4000000000014268 ) ) ;
#11462=CARTESIAN_POINT ( 'NONE',  ( 281.4928932188133786, 269.9999999999999432, 147.1999999999999886 ) ) ;
#11465=PLANE ( 'NONE',  #19971 ) ;
#11473=CARTESIAN_POINT ( 'NONE',  ( 285.1999999999999318, 267.7999999999999545, -146.4928932188133786 ) ) ;
#11480=DIRECTION ( 'NONE',  ( -1.000000000000000000, 0.000000000000000000, 0.000000000000000000 ) ) ;
#11486=AXIS2_PLACEMENT_3D ( 'NONE', #13675, #20995, #2141 ) ;
#11487=VERTEX_POINT ( 'NONE', #18472 ) ;
#11495=EDGE_LOOP ( 'NONE', ( #15192, #17731, #14327, #12492 ) ) ;
#11503=LINE ( 'NONE', #2965, #3605 ) ;
#11504=ADVANCED_FACE ( 'NONE', ( #21360 ), #8105, .F. ) ;
#11508=CARTESIAN_POINT ( 'NONE',  ( 279.9999999999999432, 273.0000000000000000, -144.9999999999999716 ) ) ;
#11509=DIRECTION ( 'NONE',  ( -3.495664435217746987E-15, 1.000000000000000000, 0.000000000000000000 ) ) ;
#11511=FACE_BOUND ( 'NONE', #17339, .T. ) ;
#11519=CARTESIAN_POINT ( 'NONE',  ( 279.9999999999999432, 273.0299999999999727, -144.9999999999999716 ) ) ;
#11527=VECTOR ( 'NONE', #1852, 1000.000000000000000 ) ;
#11529=AXIS2_PLACEMENT_3D ( 'NONE', #21338, #17717, #1174 ) ;
#11531=VECTOR ( 'NONE', #8059, 1000.000000000000000 ) ;
#11537=CARTESIAN_POINT ( 'NONE',  ( -100.0000000000001137, -129.2000000000000455, 177.2000000000014097 ) ) ;
#11539=CARTESIAN_POINT ( 'NONE',  ( -280.0000000000000568, 269.9999999999999432, 145.0000000000000284 ) ) ;
#11550=CIRCLE ( 'NONE', #9989, 2.649999999999971934 ) ;
#11551=AXIS2_PLACEMENT_3D ( 'NONE', #22212, #11156, #7608 ) ;
#11552=ADVANCED_FACE ( 'NONE', ( #15594, #22921, #13687 ), #2870, .T. ) ;
#11553=CARTESIAN_POINT ( 'NONE',  ( 281.7350371479512319, 269.1333820183295416, 145.8708543776412228 ) ) ;
#11554=DIRECTION ( 'NONE',  ( 1.000000000000000000, 0.000000000000000000, 0.000000000000000000 ) ) ;
#11558=VECTOR ( 'NONE', #17244, 1000.000000000000000 ) ;
#11560=PLANE ( 'NONE',  #14847 ) ;
#11561=DIRECTION ( 'NONE',  ( 0.000000000000000000, 0.000000000000000000, -1.000000000000000000 ) ) ;
#11564=CARTESIAN_POINT ( 'NONE',  ( 279.9999999999999432, -127.0000000000000568, 147.2000000000013813 ) ) ;
#11598=CARTESIAN_POINT ( 'NONE',  ( 281.3405375976307141, 269.5502846751311949, -145.6212670861564220 ) ) ;
#11601=ORIENTED_EDGE ( 'NONE', *, *, #1430, .F. ) ;
#11608=DIRECTION ( 'NONE',  ( 0.000000000000000000, 0.000000000000000000, 1.000000000000000000 ) ) ;
#11610=LINE ( 'NONE', #9523, #6716 ) ;
#11612=CARTESIAN_POINT ( 'NONE',  ( 281.3333820183295302, 269.5350371479512432, -145.6220388411722126 ) ) ;
#11614=FACE_BOUND ( 'NONE', #6858, .T. ) ;
#11626=DIRECTION ( 'NONE',  ( -0.000000000000000000, -0.000000000000000000, 1.000000000000000000 ) ) ;
#11643=CARTESIAN_POINT ( 'NONE',  ( -285.2000000000013529, -89.99999999999896261, -42.98333333333330586 ) ) ;
#11645=CARTESIAN_POINT ( 'NONE',  ( -281.3429506979391590, 269.5484459290825043, -145.6225751257467778 ) ) ;
#11648=CARTESIAN_POINT ( 'NONE',  ( 281.4928932188134354, -129.2000000000000455, -152.4000000000012847 ) ) ;
#11652=VERTEX_POINT ( 'NONE', #6870 ) ;
#11656=EDGE_CURVE ( 'NONE', #9824, #22116, #18251, .T. ) ;
#11660=CARTESIAN_POINT ( 'NONE',  ( 279.9999999999999432, 273.0000000000000000, -144.9999999999999716 ) ) ;
#11662=CARTESIAN_POINT ( 'NONE',  ( -281.2440776823446527, 268.3679143846943020, 147.1132285165672329 ) ) ;
#11664=ORIENTED_EDGE ( 'NONE', *, *, #21870, .F. ) ;
#11667=DIRECTION ( 'NONE',  ( 1.000000000000000000, 3.495664435217746987E-15, 0.000000000000000000 ) ) ;
#11670=CARTESIAN_POINT ( 'NONE',  ( -288.2000000000006708, 90.00000000000100897, 32.35000000000001563 ) ) ;
#11672=CARTESIAN_POINT ( 'NONE',  ( -281.4928932188134354, 267.7999999999999545, -150.1999999999999318 ) ) ;
#11677=CARTESIAN_POINT ( 'NONE',  ( -281.4928932188135491, -127.0000000000000568, 152.4000000000014268 ) ) ;
#11679=CARTESIAN_POINT ( 'NONE',  ( 279.9999999999999432, 272.9999999999999432, 145.0000000000000284 ) ) ;
#11683=CARTESIAN_POINT ( 'NONE',  ( -281.4928932188135491, -129.2000000000000455, 150.2000000000013813 ) ) ;
#11693=DIRECTION ( 'NONE',  ( -0.000000000000000000, -0.000000000000000000, -1.000000000000000000 ) ) ;
#11694=EDGE_LOOP ( 'NONE', ( #6394, #8170, #12944, #16934 ) ) ;
#11713=CARTESIAN_POINT ( 'NONE',  ( 281.7484459290825498, 269.1429506979392841, -145.8703180930665155 ) ) ;
#11717=EDGE_CURVE ( 'NONE', #4643, #8989, #13304, .T. ) ;
#11722=CARTESIAN_POINT ( 'NONE',  ( -282.2000000000010687, -19.99999999999898392, 107.6499999999999631 ) ) ;
#11726=EDGE_LOOP ( 'NONE', ( #1983, #20920, #17484, #23644 ) ) ;
#11734=CARTESIAN_POINT ( 'NONE',  ( 281.4928932188133786, 269.9999999999999432, 150.1999999999999886 ) ) ;
#11744=LINE ( 'NONE', #3851, #19097 ) ;
#11760=DIRECTION ( 'NONE',  ( -1.000000000000000000, 0.000000000000000000, -0.000000000000000000 ) ) ;
#11763=SURFACE_STYLE_FILL_AREA ( #729 ) ;
#11774=CARTESIAN_POINT ( 'NONE',  ( 283.1682701916305405, 271.9268706878665967, -145.6222583006964726 ) ) ;
#11776=CARTESIAN_POINT ( 'NONE',  ( -280.9952621458756994, 270.4339272673396977, 149.5699028110927884 ) ) ;
#11779=B_SPLINE_CURVE_WITH_KNOTS ( 'NONE', 3,
 ( #12198, #21329, #14354, #19746, #21686, #10606, #10357, #1274, #17705, #8653, #1167, #8541, #16025, #23373, #6833, #7423, #20457, #13149, #3783, #9488 ),
 .UNSPECIFIED., .F., .F.,
 ( 4, 2, 2, 2, 2, 2, 2, 2, 2, 4 ),
 ( 0.000000000000000000, 0.001035985217005822284, 0.002071970434011644567, 0.003107955651017466851, 0.003625948259520370403, 0.004143940868023274389, 0.005179926085028964400, 0.006215911302034655278, 0.007251896519040346156, 0.008287881736046037034 ),
 .UNSPECIFIED. ) ;
#11786=CARTESIAN_POINT ( 'NONE',  ( -288.2000000000008981, 35.00000000000100897, 105.0000000000000000 ) ) ;
#11788=CARTESIAN_POINT ( 'NONE',  ( -281.2440776823445390, 269.1689414351990308, -150.0938770989752697 ) ) ;
#11796=CARTESIAN_POINT ( 'NONE',  ( 281.3610889986682082, 272.8646579186752774, 145.2488155364688964 ) ) ;
#11814=LINE ( 'NONE', #14937, #6911 ) ;
#11824=LINE ( 'NONE', #17459, #5135 ) ;
#11842=VERTEX_POINT ( 'NONE', #9656 ) ;
#11876=ORIENTED_EDGE ( 'NONE', *, *, #558, .F. ) ;
#11880=CARTESIAN_POINT ( 'NONE',  ( 285.2000000000008981, 9.892604858775018348E-13, 0.000000000000000000 ) ) ;
#11883=( LENGTH_UNIT ( ) NAMED_UNIT ( * ) SI_UNIT ( .MILLI., .METRE. ) );
#11887=VECTOR ( 'NONE', #15700, 1000.000000000000000 ) ;
#11895=EDGE_CURVE ( 'NONE', #9258, #3739, #11610, .T. ) ;
#11898=CARTESIAN_POINT ( 'NONE',  ( -281.3684665762326063, 268.0840560642351988, 147.1696999999999775 ) ) ;
#11905=PLANE ( 'NONE',  #20355 ) ;
#11922=VECTOR ( 'NONE', #22632, 1000.000000000000000 ) ;
#11923=CARTESIAN_POINT ( 'NONE',  ( -45.00000000000000000, 272.9999999999999432, 5.249999999999991118 ) ) ;
#11927=FACE_OUTER_BOUND ( 'NONE', #23686, .T. ) ;
#11940=CARTESIAN_POINT ( 'NONE',  ( 34.75000000000005684, 100.0000000000000000, -147.2000000000005571 ) ) ;
#11942=CARTESIAN_POINT ( 'NONE',  ( 282.1999999999999318, 267.7999999999999545, 146.4928932188134922 ) ) ;
#11947=ORIENTED_EDGE ( 'NONE', *, *, #3655, .F. ) ;
#11954=LINE ( 'NONE', #1021, #23087 ) ;
#11966=AXIS2_PLACEMENT_3D ( 'NONE', #8747, #21302, #19466 ) ;
#11984=AXIS2_PLACEMENT_3D ( 'NONE', #3536, #20307, #3646 ) ;
#11986=AXIS2_PLACEMENT_3D ( 'NONE', #11078, #9021, #5503 ) ;
#11988=AXIS2_PLACEMENT_3D ( 'NONE', #9988, #20956, #18899 ) ;
#11990=ORIENTED_EDGE ( 'NONE', *, *, #20314, .F. ) ;
#12009=AXIS2_PLACEMENT_3D ( 'NONE', #3866, #5560, #8842 ) ;
#12025=DIRECTION ( 'NONE',  ( 0.000000000000000000, -1.000000000000000000, -5.286776307738891306E-15 ) ) ;
#12033=EDGE_CURVE ( 'NONE', #22116, #11293, #19635, .T. ) ;
#12037=ORIENTED_EDGE ( 'NONE', *, *, #21790, .F. ) ;
#12038=EDGE_CURVE ( 'NONE', #12593, #10284, #5047, .T. ) ;
#12052=LINE ( 'NONE', #988, #6581 ) ;
#12055=CARTESIAN_POINT ( 'NONE',  ( -281.3520027839448971, 269.5592670532759030, -145.6220388411722126 ) ) ;
#12063=ORIENTED_EDGE ( 'NONE', *, *, #11141, .T. ) ;
#12070=ORIENTED_EDGE ( 'NONE', *, *, #11366, .T. ) ;
#12077=FACE_OUTER_BOUND ( 'NONE', #16886, .T. ) ;
#12078=CARTESIAN_POINT ( 'NONE',  ( 45.24999999999994316, 100.0000000000000000, -147.2000000000005571 ) ) ;
#12079=ORIENTED_EDGE ( 'NONE', *, *, #12603, .T. ) ;
#12084=ORIENTED_EDGE ( 'NONE', *, *, #3808, .T. ) ;
#12089=DIRECTION ( 'NONE',  ( 0.000000000000000000, 0.000000000000000000, 1.000000000000000000 ) ) ;
#12111=VERTEX_POINT ( 'NONE', #11327 ) ;
#12117=VERTEX_POINT ( 'NONE', #8548 ) ;
#12119=LINE ( 'NONE', #10055, #18128 ) ;
#12122=EDGE_CURVE ( 'NONE', #4872, #9091, #2460, .T. ) ;
#12130=CARTESIAN_POINT ( 'NONE',  ( -40.00000000000000000, 100.0000000000000000, -150.2000000000005571 ) ) ;
#12132=FACE_OUTER_BOUND ( 'NONE', #5284, .T. ) ;
#12137=STYLED_ITEM('',(#23906),#12378);
#12138=CARTESIAN_POINT ( 'NONE',  ( -280.9952621458756994, 268.9079617568158938, 146.9223300543793584 ) ) ;
#12149=ORIENTED_EDGE ( 'NONE', *, *, #2815, .F. ) ;
#12168=EDGE_LOOP ( 'NONE', ( #1536, #2085, #4390, #4273 ) ) ;
#12171=ORIENTED_EDGE ( 'NONE', *, *, #5467, .T. ) ;
#12180=DIRECTION ( 'NONE',  ( 0.000000000000000000, 0.000000000000000000, 1.000000000000000000 ) ) ;
#12183=VERTEX_POINT ( 'NONE', #9375 ) ;
#12185=CARTESIAN_POINT ( 'NONE',  ( -287.4000000000014552, -129.2000000000000455, 146.4928932188134638 ) ) ;
#12198=CARTESIAN_POINT ( 'NONE',  ( -285.2000000000000455, 267.7999999999999545, -146.4928932188134354 ) ) ;
#12199=DIRECTION ( 'NONE',  ( 0.000000000000000000, 0.000000000000000000, 1.000000000000000000 ) ) ;
#12201=CARTESIAN_POINT ( 'NONE',  ( 287.4000000000013415, -127.0000000000000568, 146.4928932188134638 ) ) ;
#12206=DIRECTION ( 'NONE',  ( -0.000000000000000000, -1.000000000000000000, -1.110223024625156540E-16 ) ) ;
#12243=ORIENTED_EDGE ( 'NONE', *, *, #6767, .T. ) ;
#12246=DIRECTION ( 'NONE',  ( 0.000000000000000000, -0.000000000000000000, 1.000000000000000000 ) ) ;
#12248=AXIS2_PLACEMENT_3D ( 'NONE', #11045, #12636, #7037 ) ;
#12260=AXIS2_PLACEMENT_3D ( 'NONE', #7225, #2022, #14616 ) ;
#12265=LINE ( 'NONE', #23793, #8860 ) ;
#12268=EDGE_LOOP ( 'NONE', ( #5989, #21913, #21660, #3356 ) ) ;
#12274=CARTESIAN_POINT ( 'NONE',  ( -281.7350371479513456, 269.1333820183295416, -145.8708543776411659 ) ) ;
#12285=LINE ( 'NONE', #23343, #2039 ) ;
#12289=EDGE_LOOP ( 'NONE', ( #13952, #3262, #9706, #14335 ) ) ;
#12290=CARTESIAN_POINT ( 'NONE',  ( -280.9955614683503313, 270.4045710003933323, 149.5135885331258976 ) ) ;
#12297=DIRECTION ( 'NONE',  ( -0.000000000000000000, 0.000000000000000000, -1.000000000000000000 ) ) ;
#12299=DIRECTION ( 'NONE',  ( 0.000000000000000000, 1.000000000000000000, 0.000000000000000000 ) ) ;
#12308=EDGE_LOOP ( 'NONE', ( #15592, #693, #9131, #9195 ) ) ;
#12313=B_SPLINE_CURVE_WITH_KNOTS ( 'NONE', 3,
 ( #1102, #18136, #23565, #8722, #5210, #15973, #19815, #23316, #10673, #15733, #16217, #8598, #6783, #1585, #3151, #21282 ),
 .UNSPECIFIED., .F., .F.,
 ( 4, 2, 2, 2, 2, 2, 2, 4 ),
 ( 0.000000000000000000, 0.0009361184303672154955, 0.001404177645550738675, 0.001872236860734262072, 0.002340296075917785469, 0.002808355291101308649, 0.003276414506284832263, 0.003744473721468355443 ),
 .UNSPECIFIED. ) ;
#12322=EDGE_CURVE ( 'NONE', #3739, #3608, #10109, .T. ) ;
#12323=CIRCLE ( 'NONE', #2226, 5.249999999999949374 ) ;
#12327=CARTESIAN_POINT ( 'NONE',  ( -282.2000000000011255, -29.99999999999898037, -105.0000000000000000 ) ) ;
#12339=VERTEX_POINT ( 'NONE', #22980 ) ;
#12341=CARTESIAN_POINT ( 'NONE',  ( 280.8086578304521481, 269.2538215477170525, 146.6574776399288567 ) ) ;
#12342=ADVANCED_FACE ( 'NONE', ( #6452 ), #2353, .F. ) ;
#12343=VERTEX_POINT ( 'NONE', #23467 ) ;
#12365=DIRECTION ( 'NONE',  ( 0.000000000000000000, 1.000000000000000000, 0.000000000000000000 ) ) ;
#12374=EDGE_CURVE ( 'NONE', #19084, #22918, #7159, .T. ) ;
#12377=EDGE_CURVE ( 'NONE', #17025, #11293, #4883, .T. ) ;
#12378=MANIFOLD_SOLID_BREP ( 'M5 Clearance Hole1', #8697 ) ;
#12385=VERTEX_POINT ( 'NONE', #6814 ) ;
#12389=VECTOR ( 'NONE', #13786, 1000.000000000000000 ) ;
#12390=EDGE_LOOP ( 'NONE', ( #18439, #22311, #7601, #5855 ) ) ;
#12396=LINE ( 'NONE', #1458, #17704 ) ;
#12424=EDGE_LOOP ( 'NONE', ( #15134, #1874 ) ) ;
#12442=EDGE_CURVE ( 'NONE', #2692, #12111, #15500, .T. ) ;
#12445=CARTESIAN_POINT ( 'NONE',  ( -280.0000000000000568, 273.0299999999999159, 145.0000000000000284 ) ) ;
#12451=CARTESIAN_POINT ( 'NONE',  ( 285.2000000000013529, -127.0000000000000568, 146.4928932188134638 ) ) ;
#12454=DIRECTION ( 'NONE',  ( -0.000000000000000000, -1.000000000000000000, 3.495664435217746987E-15 ) ) ;
#12462=CARTESIAN_POINT ( 'NONE',  ( -282.6045710003934914, 272.3135885331261079, 145.4973317504633030 ) ) ;
#12463=VERTEX_POINT ( 'NONE', #3763 ) ;
#12466=CARTESIAN_POINT ( 'NONE',  ( 281.4301275412296945, 267.9452901038202413, 147.2000000000000171 ) ) ;
#12472=CARTESIAN_POINT ( 'NONE',  ( 280.6220388411721274, 271.9582675804705332, 148.1956429438695579 ) ) ;
#12480=EDGE_CURVE ( 'NONE', #603, #22646, #8139, .T. ) ;
#12482=EDGE_CURVE ( 'NONE', #8352, #21882, #17525, .T. ) ;
#12483=DIRECTION ( 'NONE',  ( -1.000000000000000000, 0.000000000000000000, 0.000000000000000000 ) ) ;
#12492=ORIENTED_EDGE ( 'NONE', *, *, #18547, .F. ) ;
#12493=DIRECTION ( 'NONE',  ( 0.000000000000000000, 0.000000000000000000, 1.000000000000000000 ) ) ;
#12494=ORIENTED_EDGE ( 'NONE', *, *, #21580, .T. ) ;
#12503=ADVANCED_FACE ( 'NONE', ( #21035 ), #22950, .F. ) ;
#12509=CARTESIAN_POINT ( 'NONE',  ( 285.1999999999999318, 267.7999999999999545, 0.000000000000000000 ) ) ;
#12531=CARTESIAN_POINT ( 'NONE',  ( -280.8083875057491241, 271.2314821058794223, 148.9107452280324537 ) ) ;
#12546=CARTESIAN_POINT ( 'NONE',  ( 280.2497115627124344, 269.9290760626066685, -145.5724317483736172 ) ) ;
#12547=DIRECTION ( 'NONE',  ( 1.000000000000000000, -3.495664435217746987E-15, -0.000000000000000000 ) ) ;
#12552=LINE ( 'NONE', #14231, #8349 ) ;
#12554=AXIS2_PLACEMENT_3D ( 'NONE', #1445, #22196, #5667 ) ;
#12555=ORIENTED_EDGE ( 'NONE', *, *, #20927, .T. ) ;
#12557=EDGE_LOOP ( 'NONE', ( #14648, #10149 ) ) ;
#12559=DIRECTION ( 'NONE',  ( 0.000000000000000000, -1.000000000000000000, 0.000000000000000000 ) ) ;
#12562=EDGE_CURVE ( 'NONE', #23739, #16727, #9798, .T. ) ;
#12563=VERTEX_POINT ( 'NONE', #13606 ) ;
#12565=LINE ( 'NONE', #19876, #23036 ) ;
#12567=LINE ( 'NONE', #10461, #7465 ) ;
#12575=DIRECTION ( 'NONE',  ( 0.000000000000000000, 1.000000000000000000, -3.495664435217746987E-15 ) ) ;
#12577=ORIENTED_EDGE ( 'NONE', *, *, #2839, .T. ) ;
#12583=CARTESIAN_POINT ( 'NONE',  ( 281.3684637452623747, 268.4807971656551331, 150.1999999999999886 ) ) ;
#12591=DIRECTION ( 'NONE',  ( 1.000000000000000000, 0.000000000000000000, 0.000000000000000000 ) ) ;
#12593=VERTEX_POINT ( 'NONE', #2558 ) ;
#12603=EDGE_CURVE ( 'NONE', #12593, #8982, #12313, .T. ) ;
#12613=ORIENTED_EDGE ( 'NONE', *, *, #4635, .F. ) ;
#12616=VECTOR ( 'NONE', #19984, 1000.000000000000000 ) ;
#12619=LINE ( 'NONE', #12856, #12784 ) ;
#12634=ADVANCED_FACE ( 'NONE', ( #4852, #19563, #3024, #10438 ), #17784, .F. ) ;
#12636=DIRECTION ( 'NONE',  ( -0.000000000000000000, -0.000000000000000000, 1.000000000000000000 ) ) ;
#12645=ORIENTED_EDGE ( 'NONE', *, *, #20658, .F. ) ;
#12648=DIRECTION ( 'NONE',  ( -1.000000000000000000, 3.495664435217746987E-15, 0.000000000000000000 ) ) ;
#12652=LINE ( 'NONE', #7412, #14281 ) ;
#12655=EDGE_CURVE ( 'NONE', #15403, #5390, #17115, .T. ) ;
#12656=DIRECTION ( 'NONE',  ( 1.000000000000000000, 0.000000000000000000, 0.000000000000000000 ) ) ;
#12658=AXIS2_PLACEMENT_3D ( 'NONE', #21628, #16073, #6879 ) ;
#12662=CARTESIAN_POINT ( 'NONE',  ( 281.2447782964892440, 268.3743436287469990, -147.1433523009092426 ) ) ;
#12664=CARTESIAN_POINT ( 'NONE',  ( -282.1132285165673466, 268.3679143846943020, 146.2440776823445105 ) ) ;
#12666=CARTESIAN_POINT ( 'NONE',  ( 281.0571358042175802, 270.1059783239181797, -149.6730547946946217 ) ) ;
#12688=ORIENTED_EDGE ( 'NONE', *, *, #16074, .F. ) ;
#12689=EDGE_CURVE ( 'NONE', #19505, #22159, #21987, .T. ) ;
#12706=CIRCLE ( 'NONE', #6111, 5.249999999999962697 ) ;
#12719=CIRCLE ( 'NONE', #6122, 2.649999999999971934 ) ;
#12726=CARTESIAN_POINT ( 'NONE',  ( -285.2000000000014666, -127.0000000000000568, 146.4928932188134638 ) ) ;
#12727=CARTESIAN_POINT ( 'NONE',  ( 282.1999999999999318, 267.7999999999999545, -146.4928932188133786 ) ) ;
#12730=EDGE_CURVE ( 'NONE', #5160, #22988, #11503, .T. ) ;
#12744=LINE ( 'NONE', #23564, #19654 ) ;
#12748=AXIS2_PLACEMENT_3D ( 'NONE', #13120, #9459, #15020 ) ;
#12749=CARTESIAN_POINT ( 'NONE',  ( -281.4928932188135491, -132.2000000000000455, 177.2000000000014097 ) ) ;
#12754=ORIENTED_EDGE ( 'NONE', *, *, #5772, .T. ) ;
#12778=EDGE_LOOP ( 'NONE', ( #21706, #15726, #4697, #11038 ) ) ;
#12782=AXIS2_PLACEMENT_3D ( 'NONE', #3622, #21998, #17903 ) ;
#12784=VECTOR ( 'NONE', #3504, 1000.000000000000000 ) ;
#12791=ORIENTED_EDGE ( 'NONE', *, *, #10549, .F. ) ;
#12796=DIRECTION ( 'NONE',  ( 0.000000000000000000, -1.000000000000000000, 0.000000000000000000 ) ) ;
#12800=CARTESIAN_POINT ( 'NONE',  ( -280.5758453455904942, 269.9427398886703031, 145.2488155364689248 ) ) ;
#12807=CARTESIAN_POINT ( 'NONE',  ( -282.2000000000014666, -127.0000000000000568, 146.4928932188134638 ) ) ;
#12816=DIRECTION ( 'NONE',  ( 1.000000000000000000, 0.000000000000000000, 0.000000000000000000 ) ) ;
#12820=FACE_OUTER_BOUND ( 'NONE', #5822, .T. ) ;
#12822=VERTEX_POINT ( 'NONE', #18296 ) ;
#12826=DIRECTION ( 'NONE',  ( -1.000000000000000000, -0.000000000000000000, -0.000000000000000000 ) ) ;
#12831=VERTEX_POINT ( 'NONE', #5053 ) ;
#12855=EDGE_CURVE ( 'NONE', #3554, #11487, #8664, .T. ) ;
#12856=CARTESIAN_POINT ( 'NONE',  ( -287.4000000000014552, -132.2000000000000455, -146.4928932188134070 ) ) ;
#12862=FACE_OUTER_BOUND ( 'NONE', #5221, .T. ) ;
#12871=FACE_OUTER_BOUND ( 'NONE', #9777, .T. ) ;
#12888=CYLINDRICAL_SURFACE ( 'NONE', #10604, 5.199999999999982414 ) ;
#12890=EDGE_CURVE ( 'NONE', #18256, #17025, #5154, .T. ) ;
#12899=EDGE_CURVE ( 'NONE', #21466, #18256, #12567, .T. ) ;
#12902=CARTESIAN_POINT ( 'NONE',  ( -282.2000000000000455, 268.0880230824753312, 146.3684665479255500 ) ) ;
#12904=DIRECTION ( 'NONE',  ( -6.640089860198304064E-16, -1.000000000000000000, 3.495664435217746987E-15 ) ) ;
#12905=ORIENTED_EDGE ( 'NONE', *, *, #7743, .T. ) ;
#12907=CARTESIAN_POINT ( 'NONE',  ( -281.4928932188135491, -132.2000000000000455, 152.4000000000014268 ) ) ;
#12910=VECTOR ( 'NONE', #19758, 1000.000000000000000 ) ;
#12914=CARTESIAN_POINT ( 'NONE',  ( -288.2000000000008981, 30.00000000000101963, -105.0000000000000142 ) ) ;
#12921=DIRECTION ( 'NONE',  ( -1.000000000000000000, -0.000000000000000000, -0.000000000000000000 ) ) ;
#12923=ORIENTED_EDGE ( 'NONE', *, *, #10151, .F. ) ;
#12926=CARTESIAN_POINT ( 'NONE',  ( 281.4928932188133217, -127.0000000000000568, 152.4000000000014268 ) ) ;
#12934=CARTESIAN_POINT ( 'NONE',  ( 280.9952621458755289, 270.4188186979286002, 149.5436892194421716 ) ) ;
#12940=VERTEX_POINT ( 'NONE', #1869 ) ;
#12944=ORIENTED_EDGE ( 'NONE', *, *, #4891, .T. ) ;
#12957=VERTEX_POINT ( 'NONE', #16991 ) ;
#12958=CARTESIAN_POINT ( 'NONE',  ( 281.4928932188133217, -129.2000000000000455, 152.4000000000014268 ) ) ;
#12963=CIRCLE ( 'NONE', #19079, 5.249999999999949374 ) ;
#12965=CARTESIAN_POINT ( 'NONE',  ( -285.2000000000012960, -74.99999999999899103, -90.00000000000000000 ) ) ;
#12967=ORIENTED_EDGE ( 'NONE', *, *, #20975, .T. ) ;
#12969=FACE_OUTER_BOUND ( 'NONE', #20869, .T. ) ;
#12971=CARTESIAN_POINT ( 'NONE',  ( 282.3062614524587275, 272.4728700860326853, 145.4358181722191432 ) ) ;
#12975=ORIENTED_EDGE ( 'NONE', *, *, #84, .F. ) ;
#12985=CARTESIAN_POINT ( 'NONE',  ( 281.4928932188134354, 267.8000000000000114, -147.1696999999999207 ) ) ;
#12992=CARTESIAN_POINT ( 'NONE',  ( 312.2000000000013529, -132.2000000000000455, -146.4928932188134070 ) ) ;
#13002=CARTESIAN_POINT ( 'NONE',  ( -280.4358181722192285, 272.4728700860326285, 147.3062614524587275 ) ) ;
#13004=CARTESIAN_POINT ( 'NONE',  ( -282.2000000000006708, 90.00000000000100897, 37.64999999999996305 ) ) ;
#13016=EDGE_CURVE ( 'NONE', #1301, #14664, #13693, .T. ) ;
#13042=ORIENTED_EDGE ( 'NONE', *, *, #1430, .T. ) ;
#13047=DIRECTION ( 'NONE',  ( -1.000000000000000000, 0.000000000000000000, 0.000000000000000000 ) ) ;
#13065=FACE_OUTER_BOUND ( 'NONE', #12778, .T. ) ;
#13080=CARTESIAN_POINT ( 'NONE',  ( 312.2000000000013529, -132.2000000000000455, 146.4928932188134638 ) ) ;
#13081=ORIENTED_EDGE ( 'NONE', *, *, #7252, .F. ) ;
#13094=VECTOR ( 'NONE', #1719, 1000.000000000000000 ) ;
#13095=CARTESIAN_POINT ( 'NONE',  ( 281.6810649015077388, 272.7324007871374079, 145.3120962995435832 ) ) ;
#13102=CARTESIAN_POINT ( 'NONE',  ( -282.2000000000012960, -74.99999999999899103, 90.00000000000000000 ) ) ;
#13116=CIRCLE ( 'NONE', #3020, 5.199999999999982414 ) ;
#13119=VERTEX_POINT ( 'NONE', #11940 ) ;
#13120=CARTESIAN_POINT ( 'NONE',  ( -282.2000000000006708, 90.00000000000100897, 34.99999999999999289 ) ) ;
#13134=CARTESIAN_POINT ( 'NONE',  ( -280.5743436287469308, 269.9433523009093392, 145.2481149223240777 ) ) ;
#13141=EDGE_LOOP ( 'NONE', ( #18276, #7970, #17475, #12084 ) ) ;
#13144=PLANE ( 'NONE',  #8865 ) ;
#13149=CARTESIAN_POINT ( 'NONE',  ( -280.6822561791012731, 272.9663407402829876, -145.1247002395579671 ) ) ;
#13156=ORIENTED_EDGE ( 'NONE', *, *, #23556, .T. ) ;
#13161=DIRECTION ( 'NONE',  ( -0.000000000000000000, -0.000000000000000000, 1.000000000000000000 ) ) ;
#13175=VECTOR ( 'NONE', #20238, 1000.000000000000000 ) ;
#13179=DIRECTION ( 'NONE',  ( -1.000000000000000000, -3.491481338843133355E-15, 0.000000000000000000 ) ) ;
#13181=DIRECTION ( 'NONE',  ( 0.000000000000000000, -1.000000000000000000, -5.286776307738891306E-15 ) ) ;
#13188=CARTESIAN_POINT ( 'NONE',  ( 279.9999999999999432, 272.9999999999999432, 145.0000000000000284 ) ) ;
#13192=EDGE_LOOP ( 'NONE', ( #6222, #5909, #23392, #12079 ) ) ;
#13193=CARTESIAN_POINT ( 'NONE',  ( 279.9999999999999432, 273.0299999999999159, -144.9999999999999716 ) ) ;
#13197=CARTESIAN_POINT ( 'NONE',  ( -312.2000000000014666, -132.2000000000000455, 146.4928932188134638 ) ) ;
#13203=EDGE_CURVE ( 'NONE', #8986, #12593, #19131, .T. ) ;
#13219=CARTESIAN_POINT ( 'NONE',  ( 285.1999999999998181, 268.1431883566700662, 146.4301685943532334 ) ) ;
#13228=CARTESIAN_POINT ( 'NONE',  ( 279.9999999999999432, 273.0000000000000000, -144.9999999999999716 ) ) ;
#13235=CARTESIAN_POINT ( 'NONE',  ( 284.6728700860325034, 270.1062614524586252, -146.0570750465943206 ) ) ;
#13248=DIRECTION ( 'NONE',  ( 1.000000000000000000, -0.000000000000000000, -0.000000000000000000 ) ) ;
#13250=CARTESIAN_POINT ( 'NONE',  ( -280.4976310729378497, 269.7223300543793698, -146.1079617568159392 ) ) ;
#13251=DIRECTION ( 'NONE',  ( 1.000000000000000000, 0.000000000000000000, 0.000000000000000000 ) ) ;
#13252=VERTEX_POINT ( 'NONE', #14552 ) ;
#13256=CARTESIAN_POINT ( 'NONE',  ( 281.3689414351989626, 272.8938770989752811, 145.2488155364688964 ) ) ;
#13262=ORIENTED_EDGE ( 'NONE', *, *, #3250, .T. ) ;
#13283=CARTESIAN_POINT ( 'NONE',  ( -281.4928932188135491, -127.0000000000000568, 147.2000000000013813 ) ) ;
#13285=CARTESIAN_POINT ( 'NONE',  ( 279.9999999999999432, 269.9999999999999432, -144.9999999999999716 ) ) ;
#13295=CARTESIAN_POINT ( 'NONE',  ( 280.9953931959806255, 270.4054396500290522, 149.5132312761074331 ) ) ;
#13304=CIRCLE ( 'NONE', #19022, 5.249999999999962697 ) ;
#13308=LINE ( 'NONE', #18933, #3734 ) ;
#13316=ORIENTED_EDGE ( 'NONE', *, *, #872, .T. ) ;
#13324=CARTESIAN_POINT ( 'NONE',  ( -280.2489140339770302, 272.8335297745771300, -146.3488036478619847 ) ) ;
#13326=CARTESIAN_POINT ( 'NONE',  ( 283.1755088701071941, 271.9320353020569883, 145.6228333615950419 ) ) ;
#13328=DIRECTION ( 'NONE',  ( -0.000000000000000000, 1.000000000000000000, -0.000000000000000000 ) ) ;
#13333=FACE_OUTER_BOUND ( 'NONE', #2421, .T. ) ;
#13340=CARTESIAN_POINT ( 'NONE',  ( 280.1244266708878285, 270.0000000000000000, -145.2880230824753198 ) ) ;
#13343=AXIS2_PLACEMENT_3D ( 'NONE', #1164, #2606, #15672 ) ;
#13351=EDGE_LOOP ( 'NONE', ( #9038, #9219 ) ) ;
#13362=CARTESIAN_POINT ( 'NONE',  ( -280.6220388411722411, 271.9582675804705332, -148.1956429438695579 ) ) ;
#13370=CARTESIAN_POINT ( 'NONE',  ( 282.6339272673396863, 272.3699028110927429, 145.4976310729378497 ) ) ;
#13383=DIRECTION ( 'NONE',  ( 0.000000000000000000, -1.000000000000000000, -3.495664435217746987E-15 ) ) ;
#13384=VERTEX_POINT ( 'NONE', #7772 ) ;
#13388=FACE_OUTER_BOUND ( 'NONE', #19941, .T. ) ;
#13391=DIRECTION ( 'NONE',  ( 0.000000000000000000, -3.495664435217746987E-15, 1.000000000000000000 ) ) ;
#13393=DIRECTION ( 'NONE',  ( 1.000000000000000000, -0.000000000000000000, -0.000000000000000000 ) ) ;
#13395=LINE ( 'NONE', #20341, #1284 ) ;
#13397=VERTEX_POINT ( 'NONE', #11537 ) ;
#13415=ADVANCED_FACE ( 'NONE', ( #18613 ), #12888, .T. ) ;
#13418=DIRECTION ( 'NONE',  ( 0.000000000000000000, -1.000000000000000000, 0.000000000000000000 ) ) ;
#13423=VERTEX_POINT ( 'NONE', #18515 ) ;
#13427=AXIS2_PLACEMENT_3D ( 'NONE', #11247, #3585, #1896 ) ;
#13428=ADVANCED_FACE ( 'NONE', ( #5712 ), #9470, .F. ) ;
#13429=CIRCLE ( 'NONE', #291, 2.649999999999971934 ) ;
#13432=DIRECTION ( 'NONE',  ( 1.000000000000000000, -6.938893903907227392E-16, 2.425604463963772562E-30 ) ) ;
#13440=LINE ( 'NONE', #17035, #20555 ) ;
#13447=CARTESIAN_POINT ( 'NONE',  ( 285.1999999999999318, 267.7999999999999545, 146.4928932188134922 ) ) ;
#13457=CYLINDRICAL_SURFACE ( 'NONE', #18372, 2.649999999999971934 ) ;
#13458=SHAPE_REPRESENTATION_RELATIONSHIP ( 'NONE' , 'NONE' ,  #9771, #9029 ) ;
#13463=CARTESIAN_POINT ( 'NONE',  ( 280.6220388411722411, 271.9822575857425022, -148.2140793454687469 ) ) ;
#13473=AXIS2_PLACEMENT_3D ( 'NONE', #10796, #18139, #1587 ) ;
#13481=EDGE_LOOP ( 'NONE', ( #13081, #1055, #5145, #4820 ) ) ;
#13484=CARTESIAN_POINT ( 'NONE',  ( 45.00000000000000000, 272.9999999999999432, -5.249999999999991118 ) ) ;
#13487=CARTESIAN_POINT ( 'NONE',  ( -282.2000000000000455, 267.9452901038201276, 146.4301275412297230 ) ) ;
#13493=VECTOR ( 'NONE', #10870, 1000.000000000000000 ) ;
#13497=AXIS2_PLACEMENT_3D ( 'NONE', #7952, #6138, #13906 ) ;
#13498=EDGE_CURVE ( 'NONE', #20268, #11652, #8359, .T. ) ;
#13499=CARTESIAN_POINT ( 'NONE',  ( 279.9999999999999432, 269.9696999999999889, 145.0000000000000284 ) ) ;
#13514=CARTESIAN_POINT ( 'NONE',  ( 279.9999999999999432, 272.9999999999999432, -144.9999999999999716 ) ) ;
#13528=FACE_OUTER_BOUND ( 'NONE', #11240, .T. ) ;
#13568=ORIENTED_EDGE ( 'NONE', *, *, #11176, .F. ) ;
#13577=ORIENTED_EDGE ( 'NONE', *, *, #12730, .F. ) ;
#13581=ORIENTED_EDGE ( 'NONE', *, *, #594, .F. ) ;
#13582=LINE ( 'NONE', #13806, #6535 ) ;
#13591=VERTEX_POINT ( 'NONE', #17426 ) ;
#13602=ADVANCED_FACE ( 'NONE', ( #23078 ), #4377, .F. ) ;
#13606=CARTESIAN_POINT ( 'NONE',  ( -100.0000000000001137, -132.1999999999999602, 177.2000000000014097 ) ) ;
#13611=CARTESIAN_POINT ( 'NONE',  ( -281.3684637172358975, 268.4847249064868038, -150.2299999999999613 ) ) ;
#13618=CARTESIAN_POINT ( 'NONE',  ( 284.1822575857424340, 271.0140793454687582, 145.8708543776411943 ) ) ;
#13619=CARTESIAN_POINT ( 'NONE',  ( -283.2140793454688605, 271.9822575857424454, -145.6220388411722411 ) ) ;
#13622=DIRECTION ( 'NONE',  ( -0.000000000000000000, 1.000000000000000000, -0.000000000000000000 ) ) ;
#13628=LINE ( 'NONE', #11564, #22139 ) ;
#13633=ORIENTED_EDGE ( 'NONE', *, *, #19488, .F. ) ;
#13654=CARTESIAN_POINT ( 'NONE',  ( -281.4928932188135491, -129.2000000000000455, 177.2000000000014097 ) ) ;
#13661=CARTESIAN_POINT ( 'NONE',  ( 281.4301685938040691, 268.1431883596741841, 150.1999999999999602 ) ) ;
#13662=PLANE ( 'NONE',  #23138 ) ;
#13665=CARTESIAN_POINT ( 'NONE',  ( 282.1696999999999775, 268.0840560642351988, -146.3684665762323789 ) ) ;
#13666=VECTOR ( 'NONE', #6706, 1000.000000000000000 ) ;
#13668=DIRECTION ( 'NONE',  ( -1.000000000000000000, -4.183096374613631247E-18, 0.000000000000000000 ) ) ;
#13670=DIRECTION ( 'NONE',  ( 0.000000000000000000, 0.000000000000000000, 1.000000000000000000 ) ) ;
#13675=CARTESIAN_POINT ( 'NONE',  ( -45.00000000000000000, 272.9999999999999432, 0.000000000000000000 ) ) ;
#13681=DIRECTION ( 'NONE',  ( -1.000000000000000000, -0.000000000000000000, -0.000000000000000000 ) ) ;
#13684=LINE ( 'NONE', #21003, #13736 ) ;
#13687=FACE_OUTER_BOUND ( 'NONE', #12308, .T. ) ;
#13693=CIRCLE ( 'NONE', #3221, 5.249999999999949374 ) ;
#13695=DIRECTION ( 'NONE',  ( 0.000000000000000000, 1.000000000000000000, -5.286776307738891306E-15 ) ) ;
#13700=ORIENTED_EDGE ( 'NONE', *, *, #8789, .T. ) ;
#13710=ORIENTED_EDGE ( 'NONE', *, *, #20938, .T. ) ;
#13711=CARTESIAN_POINT ( 'NONE',  ( -280.9952621458756994, 270.4188186979286002, 149.5436892194421716 ) ) ;
#13713=EDGE_LOOP ( 'NONE', ( #19277, #2821, #19556, #16026 ) ) ;
#13721=DIRECTION ( 'NONE',  ( -4.183096374613631247E-18, 1.000000000000000000, 0.000000000000000000 ) ) ;
#13730=ADVANCED_FACE ( 'NONE', ( #3027 ), #2903, .F. ) ;
#13736=VECTOR ( 'NONE', #367, 1000.000000000000000 ) ;
#13737=DIRECTION ( 'NONE',  ( 0.000000000000000000, -1.000000000000000000, 0.000000000000000000 ) ) ;
#13742=CARTESIAN_POINT ( 'NONE',  ( -285.2000000000014666, -127.0000000000000568, 146.4928932188134638 ) ) ;
#13753=ORIENTED_EDGE ( 'NONE', *, *, #15282, .T. ) ;
#13754=EDGE_CURVE ( 'NONE', #3595, #12831, #14525, .T. ) ;
#13755=EDGE_CURVE ( 'NONE', #733, #12183, #6501, .T. ) ;
#13762=FACE_OUTER_BOUND ( 'NONE', #7457, .T. ) ;
#13775=AXIS2_PLACEMENT_3D ( 'NONE', #3959, #4340, #15115 ) ;
#13778=CARTESIAN_POINT ( 'NONE',  ( 282.1427398886702917, 268.3758453455903918, -146.2440776823444537 ) ) ;
#13781=LINE ( 'NONE', #15464, #7290 ) ;
#13784=ORIENTED_EDGE ( 'NONE', *, *, #18460, .F. ) ;
#13786=DIRECTION ( 'NONE',  ( 1.000000000000000000, 3.495664435217746592E-15, -0.000000000000000000 ) ) ;
#13788=ADVANCED_FACE ( 'NONE', ( #19935 ), #8490, .F. ) ;
#13791=VERTEX_POINT ( 'NONE', #5099 ) ;
#13795=EDGE_CURVE ( 'NONE', #11293, #13591, #15867, .T. ) ;
#13806=CARTESIAN_POINT ( 'NONE',  ( -280.0000000000000568, -127.0000000000000568, -147.2000000000013245 ) ) ;
#13808=DIRECTION ( 'NONE',  ( 1.000000000000000000, -4.183096374613631247E-18, 0.000000000000000000 ) ) ;
#13810=EDGE_LOOP ( 'NONE', ( #2602, #2442, #5468, #9050 ) ) ;
#13814=AXIS2_PLACEMENT_3D ( 'NONE', #5067, #21942, #2984 ) ;
#13818=PLANE ( 'NONE',  #20215 ) ;
#13823=CARTESIAN_POINT ( 'NONE',  ( -280.1244266425809428, 269.9696999999999889, 145.2840560642350169 ) ) ;
#13829=EDGE_CURVE ( 'NONE', #13423, #1301, #5817, .T. ) ;
#13843=DIRECTION ( 'NONE',  ( -0.000000000000000000, 1.000000000000000000, -0.000000000000000000 ) ) ;
#13845=CARTESIAN_POINT ( 'NONE',  ( -282.2000000000008981, 30.00000000000101963, -105.0000000000000142 ) ) ;
#13847=CARTESIAN_POINT ( 'NONE',  ( -281.3610889986683219, 272.8646579186752774, -145.2488155364688396 ) ) ;
#13856=ORIENTED_EDGE ( 'NONE', *, *, #1516, .F. ) ;
#13857=LINE ( 'NONE', #18884, #9445 ) ;
#13892=ADVANCED_FACE ( 'NONE', ( #3511 ), #3738, .F. ) ;
#13906=DIRECTION ( 'NONE',  ( -6.640089860198304064E-16, -1.000000000000000000, 0.000000000000000000 ) ) ;
#13911=CARTESIAN_POINT ( 'NONE',  ( -280.8086578304520913, 269.2538215477169388, -146.6574776399288282 ) ) ;
#13915=VECTOR ( 'NONE', #1123, 1000.000000000000000 ) ;
#13917=AXIS2_PLACEMENT_3D ( 'NONE', #10100, #11561, #2578 ) ;
#13932=DIRECTION ( 'NONE',  ( -3.700743415417188731E-15, -1.000000000000000000, -0.000000000000000000 ) ) ;
#13938=DIRECTION ( 'NONE',  ( -0.000000000000000000, 0.000000000000000000, -1.000000000000000000 ) ) ;
#13952=ORIENTED_EDGE ( 'NONE', *, *, #19297, .F. ) ;
#13956=FACE_OUTER_BOUND ( 'NONE', #19940, .T. ) ;
#13958=VERTEX_POINT ( 'NONE', #1938 ) ;
#13970=ADVANCED_FACE ( 'NONE', ( #12862 ), #20167, .T. ) ;
#13975=CARTESIAN_POINT ( 'NONE',  ( -282.1697000000000912, 267.7999999999999545, -146.4928932188134354 ) ) ;
#13990=CARTESIAN_POINT ( 'NONE',  ( 280.2906609804447839, 269.9854425596107603, 145.1255802622536919 ) ) ;
#14014=ADVANCED_FACE ( 'NONE', ( #15242 ), #21132, .F. ) ;
#14019=CARTESIAN_POINT ( 'NONE',  ( -280.6212670861564789, 269.5502846751312518, -146.3405375976306573 ) ) ;
#14024=ADVANCED_FACE ( 'NONE', ( #4476 ), #2415, .T. ) ;
#14026=CARTESIAN_POINT ( 'NONE',  ( 280.2488155364687827, 272.8938770989752811, 146.3689414351990763 ) ) ;
#14029=CARTESIAN_POINT ( 'NONE',  ( -287.4000000000014552, -129.2000000000000455, 146.4928932188134638 ) ) ;
#14030=EDGE_CURVE ( 'NONE', #3613, #8918, #6286, .T. ) ;
#14040=CARTESIAN_POINT ( 'NONE',  ( -288.2000000000006708, 90.00000000000100897, 37.64999999999996305 ) ) ;
#14047=ADVANCED_FACE ( 'NONE', ( #19070 ), #4351, .F. ) ;
#14048=ORIENTED_EDGE ( 'NONE', *, *, #13016, .T. ) ;
#14049=CYLINDRICAL_SURFACE ( 'NONE', #15315, 5.249999999999942268 ) ;
#14055=EDGE_CURVE ( 'NONE', #22842, #20948, #2269, .T. ) ;
#14058=CARTESIAN_POINT ( 'NONE',  ( -285.2000000000010687, -19.99999999999898392, 105.0000000000000000 ) ) ;
#14070=VERTEX_POINT ( 'NONE', #11648 ) ;
#14071=ORIENTED_EDGE ( 'NONE', *, *, #2025, .T. ) ;
#14076=CARTESIAN_POINT ( 'NONE',  ( 287.4000000000013415, -127.0000000000000568, -146.4928932188134070 ) ) ;
#14078=EDGE_CURVE ( 'NONE', #20948, #4643, #4097, .T. ) ;
#14082=EDGE_CURVE ( 'NONE', #10936, #4595, #18826, .T. ) ;
#14085=CARTESIAN_POINT ( 'NONE',  ( -282.2000000000008981, 30.00000000000101963, -102.3500000000000369 ) ) ;
#14090=EDGE_CURVE ( 'NONE', #21882, #12343, #6039, .T. ) ;
#14104=EDGE_LOOP ( 'NONE', ( #18261, #23801, #8530, #16043, #2172, #15831, #16346, #15408 ) ) ;
#14109=CARTESIAN_POINT ( 'NONE',  ( -288.2000000000011255, -29.99999999999898037, -102.3500000000000227 ) ) ;
#14117=DIRECTION ( 'NONE',  ( -1.000000000000000000, 0.000000000000000000, 0.000000000000000000 ) ) ;
#14120=VECTOR ( 'NONE', #15322, 1000.000000000000000 ) ;
#14125=LINE ( 'NONE', #17718, #9281 ) ;
#14131=CIRCLE ( 'NONE', #18655, 5.199999999999982414 ) ;
#14141=CARTESIAN_POINT ( 'NONE',  ( 280.4976310729377360, 272.3699028110927429, 147.6339272673398284 ) ) ;
#14146=AXIS2_PLACEMENT_3D ( 'NONE', #22724, #15264, #18852 ) ;
#14150=VERTEX_POINT ( 'NONE', #2249 ) ;
#14154=ADVANCED_FACE ( 'NONE', ( #7452 ), #3827, .F. ) ;
#14166=CIRCLE ( 'NONE', #3709, 5.199999999999982414 ) ;
#14168=ORIENTED_EDGE ( 'NONE', *, *, #18957, .F. ) ;
#14169=DIRECTION ( 'NONE',  ( 0.000000000000000000, -3.495664435217746987E-15, 1.000000000000000000 ) ) ;
#14176=AXIS2_PLACEMENT_3D ( 'NONE', #13102, #18708, #16685 ) ;
#14184=ORIENTED_EDGE ( 'NONE', *, *, #21870, .T. ) ;
#14189=CARTESIAN_POINT ( 'NONE',  ( -40.00000000000000000, 100.0000000000000000, 150.2000000000009550 ) ) ;
#14190=CARTESIAN_POINT ( 'NONE',  ( -280.5679143846944044, 269.9132285165672442, -145.2488155364688396 ) ) ;
#14201=CARTESIAN_POINT ( 'NONE',  ( 285.1999999999999318, 267.7999999999999545, -146.4928932188133786 ) ) ;
#14208=CARTESIAN_POINT ( 'NONE',  ( 35.00000000000000711, -3.880967142342036772E-28, -147.2000000000008981 ) ) ;
#14213=CIRCLE ( 'NONE', #23540, 5.199999999999982414 ) ;
#14216=ORIENTED_EDGE ( 'NONE', *, *, #2643, .F. ) ;
#14222=EDGE_LOOP ( 'NONE', ( #13577, #18084, #4470, #21630 ) ) ;
#14224=AXIS2_PLACEMENT_3D ( 'NONE', #1356, #16100, #5224 ) ;
#14230=CARTESIAN_POINT ( 'NONE',  ( -282.1697000000000912, 268.0840560642351988, 146.3684665762324357 ) ) ;
#14231=CARTESIAN_POINT ( 'NONE',  ( 279.9999999999999432, 269.9999999999999432, -144.9999999999999716 ) ) ;
#14237=PLANE ( 'NONE',  #23076 ) ;
#14246=FACE_OUTER_BOUND ( 'NONE', #15418, .T. ) ;
#14250=CARTESIAN_POINT ( 'NONE',  ( -281.6795879751485359, 272.7329465209280102, 145.3118087683467934 ) ) ;
#14254=CARTESIAN_POINT ( 'NONE',  ( 280.1255313583545785, 270.0000000000000568, 145.2905802150185650 ) ) ;
#14262=VECTOR ( 'NONE', #13622, 1000.000000000000000 ) ;
#14265=CARTESIAN_POINT ( 'NONE',  ( 281.3684637172357270, 268.4847249064869743, 150.2299999999999898 ) ) ;
#14274=EDGE_LOOP ( 'NONE', ( #8604, #23359 ) ) ;
#14281=VECTOR ( 'NONE', #21781, 1000.000000000000000 ) ;
#14286=CARTESIAN_POINT ( 'NONE',  ( -288.2000000000011255, -29.99999999999898037, -105.0000000000000000 ) ) ;
#14295=AXIS2_PLACEMENT_3D ( 'NONE', #6332, #16000, #8628 ) ;
#14300=EDGE_LOOP ( 'NONE', ( #9018, #5826 ) ) ;
#14304=DIRECTION ( 'NONE',  ( 0.000000000000000000, -1.000000000000000000, -3.495664435217746987E-15 ) ) ;
#14317=ORIENTED_EDGE ( 'NONE', *, *, #23692, .F. ) ;
#14320=CARTESIAN_POINT ( 'NONE',  ( 281.4928932188134354, 267.8000000000000114, -150.2299999999999329 ) ) ;
#14323=CARTESIAN_POINT ( 'NONE',  ( 281.4928932188134354, -127.0000000000000568, -152.4000000000012847 ) ) ;
#14327=ORIENTED_EDGE ( 'NONE', *, *, #15714, .T. ) ;
#14335=ORIENTED_EDGE ( 'NONE', *, *, #11316, .F. ) ;
#14336=CARTESIAN_POINT ( 'NONE',  ( -281.0571358042176939, 270.1059783239181797, 149.6730547946947354 ) ) ;
#14348=DIRECTION ( 'NONE',  ( -0.000000000000000000, -1.000000000000000000, 6.123233995736766036E-17 ) ) ;
#14351=CARTESIAN_POINT ( 'NONE',  ( -281.9223300543794721, 268.9079617568158938, 145.9952621458756425 ) ) ;
#14354=CARTESIAN_POINT ( 'NONE',  ( -285.1663417894422992, 268.4816199723480281, -146.3683070494394940 ) ) ;
#14359=EDGE_LOOP ( 'NONE', ( #21489, #2787, #21678, #1211 ) ) ;
#14361=CARTESIAN_POINT ( 'NONE',  ( -281.4928932188134354, -132.2000000000000455, -177.2000000000013529 ) ) ;
#14366=CARTESIAN_POINT ( 'NONE',  ( 7.690461757479017101E-15, -129.2000000000000455, 0.000000000000000000 ) ) ;
#14367=DIRECTION ( 'NONE',  ( 1.000000000000000000, 0.000000000000000000, -0.000000000000000000 ) ) ;
#14370=CARTESIAN_POINT ( 'NONE',  ( -285.2000000000006708, 90.00000000000102318, -35.00000000000001421 ) ) ;
#14386=LINE ( 'NONE', #20019, #14967 ) ;
#14402=PLANE ( 'NONE',  #3659 ) ;
#14403=CARTESIAN_POINT ( 'NONE',  ( 285.2000000000013529, -127.0000000000000568, -146.4928932188134070 ) ) ;
#14411=DIRECTION ( 'NONE',  ( -0.000000000000000000, -0.000000000000000000, 1.000000000000000000 ) ) ;
#14414=DIRECTION ( 'NONE',  ( 0.000000000000000000, -0.000000000000000000, 1.000000000000000000 ) ) ;
#14416=FACE_OUTER_BOUND ( 'NONE', #632, .T. ) ;
#14421=DIRECTION ( 'NONE',  ( -6.640089860198304064E-16, -1.000000000000000000, 3.495664435217746987E-15 ) ) ;
#14424=DIRECTION ( 'NONE',  ( 3.495664435217746987E-15, 1.000000000000000000, 0.000000000000000000 ) ) ;
#14433=ORIENTED_EDGE ( 'NONE', *, *, #5471, .F. ) ;
#14435=DIRECTION ( 'NONE',  ( 0.000000000000000000, 0.000000000000000000, 1.000000000000000000 ) ) ;
#14455=CARTESIAN_POINT ( 'NONE',  ( 281.1810844504668125, 269.4795879751484904, -149.9329465209279704 ) ) ;
#14462=ORIENTED_EDGE ( 'NONE', *, *, #4184, .T. ) ;
#14472=CIRCLE ( 'NONE', #21732, 5.249999999999962697 ) ;
#14484=CYLINDRICAL_SURFACE ( 'NONE', #23685, 5.199999999999982414 ) ;
#14486=ORIENTED_EDGE ( 'NONE', *, *, #19719, .F. ) ;
#14489=VERTEX_POINT ( 'NONE', #3093 ) ;
#14494=CARTESIAN_POINT ( 'NONE',  ( 285.2299999999999045, 267.7999999999999545, -146.4928932188133786 ) ) ;
#14495=VECTOR ( 'NONE', #11217, 1000.000000000000000 ) ;
#14512=EDGE_CURVE ( 'NONE', #3355, #12111, #8542, .T. ) ;
#14513=ORIENTED_EDGE ( 'NONE', *, *, #20938, .F. ) ;
#14520=CARTESIAN_POINT ( 'NONE',  ( -287.4000000000014552, -132.2000000000000455, -146.4928932188134070 ) ) ;
#14525=LINE ( 'NONE', #4979, #2657 ) ;
#14552=CARTESIAN_POINT ( 'NONE',  ( 35.00000000000000711, -3.880967142342036772E-28, -150.2000000000008981 ) ) ;
#14553=FACE_OUTER_BOUND ( 'NONE', #7466, .T. ) ;
#14561=CARTESIAN_POINT ( 'NONE',  ( 280.9954397628184779, 268.9021437883073986, -146.9094021484633856 ) ) ;
#14565=DIRECTION ( 'NONE',  ( 1.000000000000000000, -3.495664435217746987E-15, -0.000000000000000000 ) ) ;
#14567=CARTESIAN_POINT ( 'NONE',  ( 280.4358181722191148, 272.4728700860325148, -147.3062614524586138 ) ) ;
#14576=FACE_BOUND ( 'NONE', #14953, .T. ) ;
#14586=DIRECTION ( 'NONE',  ( 0.000000000000000000, 0.000000000000000000, -1.000000000000000000 ) ) ;
#14588=DIRECTION ( 'NONE',  ( 1.000000000000000000, -0.000000000000000000, -0.000000000000000000 ) ) ;
#14591=LINE ( 'NONE', #21939, #168 ) ;
#14603=DIRECTION ( 'NONE',  ( 0.000000000000000000, -1.000000000000000000, 0.000000000000000000 ) ) ;
#14616=DIRECTION ( 'NONE',  ( 0.000000000000000000, -1.000000000000000000, 0.000000000000000000 ) ) ;
#14633=EDGE_CURVE ( 'NONE', #22322, #8986, #22873, .T. ) ;
#14646=CIRCLE ( 'NONE', #20826, 2.199999999999979750 ) ;
#14648=ORIENTED_EDGE ( 'NONE', *, *, #23777, .F. ) ;
#14660=ORIENTED_EDGE ( 'NONE', *, *, #16709, .F. ) ;
#14663=DIRECTION ( 'NONE',  ( -4.183096374613631247E-18, 1.000000000000000000, 0.000000000000000000 ) ) ;
#14664=VERTEX_POINT ( 'NONE', #8562 ) ;
#14682=EDGE_CURVE ( 'NONE', #19104, #13591, #22908, .T. ) ;
#14689=CARTESIAN_POINT ( 'NONE',  ( 281.4928932188134354, 267.8000000000000114, -144.9999999999999716 ) ) ;
#14695=CARTESIAN_POINT ( 'NONE',  ( -282.1427398886704054, 268.3758453455903918, 146.2440776823445105 ) ) ;
#14699=VERTEX_POINT ( 'NONE', #3807 ) ;
#14706=FACE_BOUND ( 'NONE', #14274, .T. ) ;
#14721=CARTESIAN_POINT ( 'NONE',  ( 281.3684665762323789, 268.0840560642351988, 147.1696999999999775 ) ) ;
#14724=ORIENTED_EDGE ( 'NONE', *, *, #787, .T. ) ;
#14746=CARTESIAN_POINT ( 'NONE',  ( -40.00000000000000000, 100.0000000000000000, -147.2000000000005571 ) ) ;
#14757=CARTESIAN_POINT ( 'NONE',  ( -282.1433523009093847, 268.3743436287468853, -146.2447782964893577 ) ) ;
#14760=DIRECTION ( 'NONE',  ( -0.000000000000000000, -0.000000000000000000, 1.000000000000000000 ) ) ;
#14770=CARTESIAN_POINT ( 'NONE',  ( 280.8708543776411943, 269.1333820183295984, -146.7350371479512887 ) ) ;
#14772=ORIENTED_EDGE ( 'NONE', *, *, #22749, .T. ) ;
#14779=CARTESIAN_POINT ( 'NONE',  ( 287.4000000000013415, -127.0000000000000568, 146.4928932188134638 ) ) ;
#14792=CARTESIAN_POINT ( 'NONE',  ( -281.4928932188134922, 269.9999999999999432, -150.1999999999999318 ) ) ;
#14798=ADVANCED_FACE ( 'NONE', ( #1651 ), #20346, .F. ) ;
#14802=EDGE_LOOP ( 'NONE', ( #3001, #5604, #9636, #2784 ) ) ;
#14803=CARTESIAN_POINT ( 'NONE',  ( 280.8089314698394219, 269.2533442688713876, -146.6578961534456198 ) ) ;
#14807=EDGE_CURVE ( 'NONE', #21417, #10987, #7197, .T. ) ;
#14811=EDGE_LOOP ( 'NONE', ( #20185, #2908, #6025, #20976 ) ) ;
#14815=DIRECTION ( 'NONE',  ( -3.495664435217746987E-15, -1.000000000000000000, 0.000000000000000000 ) ) ;
#14829=CARTESIAN_POINT ( 'NONE',  ( -285.2000000000010118, 9.892604858775022387E-13, 146.4928932188134638 ) ) ;
#14834=FACE_OUTER_BOUND ( 'NONE', #19052, .T. ) ;
#14837=VERTEX_POINT ( 'NONE', #18087 ) ;
#14840=EDGE_CURVE ( 'NONE', #5337, #8352, #1999, .T. ) ;
#14847=AXIS2_PLACEMENT_3D ( 'NONE', #9848, #1981, #2343 ) ;
#14863=FACE_OUTER_BOUND ( 'NONE', #8830, .T. ) ;
#14864=AXIS2_PLACEMENT_3D ( 'NONE', #7596, #14989, #17144 ) ;
#14877=CARTESIAN_POINT ( 'NONE',  ( 284.5135885331259260, 270.4045710003932754, 145.9955614683503313 ) ) ;
#14881=FACE_BOUND ( 'NONE', #6780, .T. ) ;
#14884=ORIENTED_EDGE ( 'NONE', *, *, #20858, .T. ) ;
#14898=DIRECTION ( 'NONE',  ( -3.700743415417188731E-15, -1.000000000000000000, -0.000000000000000000 ) ) ;
#14900=ADVANCED_FACE ( 'NONE', ( #15310 ), #22411, .F. ) ;
#14914=DIRECTION ( 'NONE',  ( 0.000000000000000000, 0.000000000000000000, 1.000000000000000000 ) ) ;
#14923=LINE ( 'NONE', #18525, #17153 ) ;
#14926=LINE ( 'NONE', #20211, #18867 ) ;
#14936=ORIENTED_EDGE ( 'NONE', *, *, #12655, .T. ) ;
#14937=CARTESIAN_POINT ( 'NONE',  ( 287.4000000000013415, -129.2000000000000455, -146.4928932188134070 ) ) ;
#14940=DIRECTION ( 'NONE',  ( 1.000000000000000000, -3.495664435217746592E-15, 0.000000000000000000 ) ) ;
#14944=DIRECTION ( 'NONE',  ( -0.000000000000000000, -0.000000000000000000, 1.000000000000000000 ) ) ;
#14945=CIRCLE ( 'NONE', #12658, 2.649999999999971934 ) ;
#14953=EDGE_LOOP ( 'NONE', ( #13633, #20835 ) ) ;
#14964=FACE_OUTER_BOUND ( 'NONE', #211, .T. ) ;
#14967=VECTOR ( 'NONE', #18214, 1000.000000000000000 ) ;
#14969=CARTESIAN_POINT ( 'NONE',  ( 283.1956429438695295, 271.9582675804705332, -145.6220388411722126 ) ) ;
#14977=EDGE_LOOP ( 'NONE', ( #15014, #15130, #20793, #3233 ) ) ;
#14985=DIRECTION ( 'NONE',  ( 0.000000000000000000, -1.000000000000000000, 0.000000000000000000 ) ) ;
#14989=DIRECTION ( 'NONE',  ( -1.000000000000000000, 3.495664435217746987E-15, 0.000000000000000000 ) ) ;
#14990=VERTEX_POINT ( 'NONE', #22520 ) ;
#14992=LINE ( 'NONE', #11271, #22919 ) ;
#14994=CARTESIAN_POINT ( 'NONE',  ( -285.2000000000012960, -74.99999999999899103, -90.00000000000000000 ) ) ;
#14995=DIRECTION ( 'NONE',  ( 0.000000000000000000, 0.000000000000000000, -1.000000000000000000 ) ) ;
#14999=FACE_OUTER_BOUND ( 'NONE', #11495, .T. ) ;
#15014=ORIENTED_EDGE ( 'NONE', *, *, #62, .F. ) ;
#15016=CARTESIAN_POINT ( 'NONE',  ( 285.1663407402830899, 268.4822561791008866, -146.3681929792553547 ) ) ;
#15020=DIRECTION ( 'NONE',  ( 0.000000000000000000, -1.000000000000000000, 0.000000000000000000 ) ) ;
#15021=DIRECTION ( 'NONE',  ( 1.000000000000000000, 0.000000000000000000, 0.000000000000000000 ) ) ;
#15024=CARTESIAN_POINT ( 'NONE',  ( -282.2000000000013529, -89.99999999999897682, 21.68333333333335844 ) ) ;
#15035=AXIS2_PLACEMENT_3D ( 'NONE', #18271, #167, #19854 ) ;
#15036=CARTESIAN_POINT ( 'NONE',  ( -280.4976310729378497, 269.6958543268121957, -146.0927021017107279 ) ) ;
#15048=CARTESIAN_POINT ( 'NONE',  ( 283.2140793454687469, 271.9822575857424454, 145.6220388411722979 ) ) ;
#15049=CARTESIAN_POINT ( 'NONE',  ( -280.0000000000000568, 273.0299999999999159, -144.9999999999999716 ) ) ;
#15058=AXIS2_PLACEMENT_3D ( 'NONE', #128, #3379, #18135 ) ;
#15076=CARTESIAN_POINT ( 'NONE',  ( 281.4928932188133217, 267.7999999999999545, 147.1999999999999886 ) ) ;
#15093=CARTESIAN_POINT ( 'NONE',  ( 280.4973317504630472, 272.3135885331258805, 147.6045710003933777 ) ) ;
#15111=ORIENTED_EDGE ( 'NONE', *, *, #11176, .T. ) ;
#15112=CARTESIAN_POINT ( 'NONE',  ( -288.2000000000008981, 35.00000000000100897, 102.3500000000000227 ) ) ;
#15115=DIRECTION ( 'NONE',  ( 0.000000000000000000, 0.000000000000000000, 1.000000000000000000 ) ) ;
#15118=CARTESIAN_POINT ( 'NONE',  ( 99.99999999999994316, 4.509448885211231533E-13, 150.2000000000009550 ) ) ;
#15124=CARTESIAN_POINT ( 'NONE',  ( -280.5908103165960483, 272.0295083325148653, -148.0299054689546665 ) ) ;
#15126=DIRECTION ( 'NONE',  ( 1.000000000000000000, -3.495664435217746987E-15, -0.000000000000000000 ) ) ;
#15130=ORIENTED_EDGE ( 'NONE', *, *, #4795, .T. ) ;
#15131=DIRECTION ( 'NONE',  ( -1.000000000000000000, -0.000000000000000000, -0.000000000000000000 ) ) ;
#15133=ORIENTED_EDGE ( 'NONE', *, *, #22088, .F. ) ;
#15134=ORIENTED_EDGE ( 'NONE', *, *, #9299, .F. ) ;
#15136=CARTESIAN_POINT ( 'NONE',  ( 281.2440776823445390, 269.1610889986682764, -150.0646579186751808 ) ) ;
#15145=VERTEX_POINT ( 'NONE', #8642 ) ;
#15153=DIRECTION ( 'NONE',  ( 1.000000000000000000, 0.000000000000000000, 0.000000000000000000 ) ) ;
#15155=CARTESIAN_POINT ( 'NONE',  ( -281.3684665479255500, 268.0880230824753312, -147.1999999999999318 ) ) ;
#15158=PLANE ( 'NONE',  #20421 ) ;
#15160=DIRECTION ( 'NONE',  ( 0.000000000000000000, 0.000000000000000000, 1.000000000000000000 ) ) ;
#15164=AXIS2_PLACEMENT_3D ( 'NONE', #11734, #11480, #13670 ) ;
#15178=VERTEX_POINT ( 'NONE', #7168 ) ;
#15192=ORIENTED_EDGE ( 'NONE', *, *, #12899, .T. ) ;
#15195=LINE ( 'NONE', #5769, #17536 ) ;
#15198=ORIENTED_EDGE ( 'NONE', *, *, #18957, .T. ) ;
#15202=ORIENTED_EDGE ( 'NONE', *, *, #313, .F. ) ;
#15209=CARTESIAN_POINT ( 'NONE',  ( 282.1132285165672329, 268.3679143846943020, -146.2440776823444537 ) ) ;
#15210=FACE_BOUND ( 'NONE', #19659, .T. ) ;
#15215=ADVANCED_FACE ( 'NONE', ( #18174 ), #20098, .F. ) ;
#15219=CARTESIAN_POINT ( 'NONE',  ( -34.75000000000005684, 100.0000000000000000, -150.2000000000005571 ) ) ;
#15221=EDGE_CURVE ( 'NONE', #8352, #22022, #10953, .T. ) ;
#15223=FACE_OUTER_BOUND ( 'NONE', #13481, .T. ) ;
#15242=FACE_OUTER_BOUND ( 'NONE', #22310, .T. ) ;
#15250=CARTESIAN_POINT ( 'NONE',  ( 281.2440776823445390, 269.1689414351990308, -150.0938770989752413 ) ) ;
#15254=AXIS2_PLACEMENT_3D ( 'NONE', #22527, #20860, #13181 ) ;
#15264=DIRECTION ( 'NONE',  ( 0.000000000000000000, -3.495664435217746987E-15, -1.000000000000000000 ) ) ;
#15266=CARTESIAN_POINT ( 'NONE',  ( -45.00000000000000000, 269.9999999999999432, 0.000000000000000000 ) ) ;
#15273=CARTESIAN_POINT ( 'NONE',  ( -280.2488155364688964, 272.8646579186752774, -146.3610889986682650 ) ) ;
#15276=ORIENTED_EDGE ( 'NONE', *, *, #14090, .F. ) ;
#15282=EDGE_CURVE ( 'NONE', #12463, #5386, #1974, .T. ) ;
#15283=CARTESIAN_POINT ( 'NONE',  ( 285.0938770989752697, 269.1689414351989740, 146.2440776823445958 ) ) ;
#15285=LINE ( 'NONE', #177, #16825 ) ;
#15291=FACE_OUTER_BOUND ( 'NONE', #13810, .T. ) ;
#15299=VERTEX_POINT ( 'NONE', #22493 ) ;
#15301=CARTESIAN_POINT ( 'NONE',  ( -281.4928932188134922, 267.7999999999999545, 147.1999999999999886 ) ) ;
#15310=FACE_OUTER_BOUND ( 'NONE', #4151, .T. ) ;
#15315=AXIS2_PLACEMENT_3D ( 'NONE', #15854, #21378, #10069 ) ;
#15316=CARTESIAN_POINT ( 'NONE',  ( 45.00000000000000000, 269.9999999999999432, -5.249999999999973355 ) ) ;
#15322=DIRECTION ( 'NONE',  ( -1.000000000000000000, 3.495664435217746592E-15, -0.000000000000000000 ) ) ;
#15323=LINE ( 'NONE', #17015, #19212 ) ;
#15324=VERTEX_POINT ( 'NONE', #9479 ) ;
#15326=CARTESIAN_POINT ( 'NONE',  ( 282.1999999999999318, 268.0880230824753312, -146.3684665479254932 ) ) ;
#15329=PLANE ( 'NONE',  #8907 ) ;
#15345=LINE ( 'NONE', #5905, #2897 ) ;
#15363=VECTOR ( 'NONE', #1950, 1000.000000000000000 ) ;
#15372=EDGE_CURVE ( 'NONE', #13252, #22418, #769, .T. ) ;
#15375=ORIENTED_EDGE ( 'NONE', *, *, #16074, .T. ) ;
#15389=CARTESIAN_POINT ( 'NONE',  ( -280.9952621458755857, 270.4339272673397545, -149.5699028110927600 ) ) ;
#15401=CARTESIAN_POINT ( 'NONE',  ( 279.9999999999999432, 269.9999999999999432, 145.0000000000000284 ) ) ;
#15402=CARTESIAN_POINT ( 'NONE',  ( -284.5699028110928452, 270.4339272673396977, -145.9952621458756141 ) ) ;
#15403=VERTEX_POINT ( 'NONE', #22965 ) ;
#15408=ORIENTED_EDGE ( 'NONE', *, *, #6365, .T. ) ;
#15418=EDGE_LOOP ( 'NONE', ( #14184, #15375, #17810, #2278 ) ) ;
#15420=ADVANCED_FACE ( 'NONE', ( #10197 ), #4508, .F. ) ;
#15423=ORIENTED_EDGE ( 'NONE', *, *, #8894, .F. ) ;
#15426=VECTOR ( 'NONE', #15602, 1000.000000000000000 ) ;
#15438=EDGE_LOOP ( 'NONE', ( #18578, #20437 ) ) ;
#15448=ORIENTED_EDGE ( 'NONE', *, *, #8789, .F. ) ;
#15453=CARTESIAN_POINT ( 'NONE',  ( 280.4357574145958552, 272.4730547946948036, 147.3059783239181115 ) ) ;
#15455=EDGE_CURVE ( 'NONE', #5390, #9249, #12052, .T. ) ;
#15461=CARTESIAN_POINT ( 'NONE',  ( -281.4928932188134354, -127.0000000000000568, -152.4000000000012847 ) ) ;
#15462=CARTESIAN_POINT ( 'NONE',  ( -280.0000000000000568, 269.9999999999999432, 145.0000000000000284 ) ) ;
#15464=CARTESIAN_POINT ( 'NONE',  ( 312.2000000000013529, -132.2000000000000455, 0.000000000000000000 ) ) ;
#15467=AXIS2_PLACEMENT_3D ( 'NONE', #15921, #23257, #4443 ) ;
#15473=CYLINDRICAL_SURFACE ( 'NONE', #20997, 2.199999999999979750 ) ;
#15481=CARTESIAN_POINT ( 'NONE',  ( 312.2000000000013529, -132.2000000000000455, -146.4928932188134070 ) ) ;
#15488=DIRECTION ( 'NONE',  ( -1.000000000000000000, 0.000000000000000000, 0.000000000000000000 ) ) ;
#15489=CARTESIAN_POINT ( 'NONE',  ( -281.4928932188135491, -129.2000000000000455, 177.2000000000014097 ) ) ;
#15490=ORIENTED_EDGE ( 'NONE', *, *, #23146, .T. ) ;
#15492=( NAMED_UNIT ( * ) SI_UNIT ( $, .STERADIAN. ) SOLID_ANGLE_UNIT ( ) );
#15500=B_SPLINE_CURVE_WITH_KNOTS ( 'NONE', 3,
 ( #8631, #8758, #8522, #16119, #21420, #14336, #12290, #21665, #5123, #12531, #22239, #18728, #5591, #9466, #13002, #16818, #5356, #5837, #22117, #20303 ),
 .UNSPECIFIED., .F., .F.,
 ( 4, 2, 2, 2, 2, 2, 2, 2, 2, 4 ),
 ( 0.000000000000000000, 0.001035985217005782819, 0.002071970434011565637, 0.003107955651017348889, 0.003625948259520284968, 0.004143940868023221480, 0.005179926085028920164, 0.006215911302034618849, 0.007251896519040319268, 0.008287881736046017953 ),
 .UNSPECIFIED. ) ;
#15504=CARTESIAN_POINT ( 'NONE',  ( -280.4976310729379065, 269.7223300543793698, 146.1079617568159961 ) ) ;
#15518=ORIENTED_EDGE ( 'NONE', *, *, #2839, .F. ) ;
#15523=EDGE_CURVE ( 'NONE', #4045, #13958, #21869, .T. ) ;
#15525=CARTESIAN_POINT ( 'NONE',  ( -280.2840560642353012, 269.9696999999999889, -145.1244266425809712 ) ) ;
#15533=VECTOR ( 'NONE', #3937, 1000.000000000000000 ) ;
#15534=DIRECTION ( 'NONE',  ( 0.000000000000000000, -1.000000000000000000, 6.123233995736766036E-17 ) ) ;
#15545=ADVANCED_FACE ( 'NONE', ( #12871 ), #10809, .F. ) ;
#15553=CARTESIAN_POINT ( 'NONE',  ( -287.4000000000014552, -127.0000000000000568, 146.4928932188134638 ) ) ;
#15559=CARTESIAN_POINT ( 'NONE',  ( 40.00000000000000000, 100.0000000000000000, 150.2000000000009550 ) ) ;
#15562=PLANE ( 'NONE',  #13343 ) ;
#15566=EDGE_LOOP ( 'NONE', ( #14168, #8340, #5415, #8559 ) ) ;
#15577=ORIENTED_EDGE ( 'NONE', *, *, #19488, .T. ) ;
#15582=AXIS2_PLACEMENT_3D ( 'NONE', #22209, #3971, #22340 ) ;
#15586=EDGE_LOOP ( 'NONE', ( #16459, #4098, #4694, #2468 ) ) ;
#15587=CARTESIAN_POINT ( 'NONE',  ( 280.1244295015774810, 273.0299999999999159, 145.6847249064867356 ) ) ;
#15592=ORIENTED_EDGE ( 'NONE', *, *, #4889, .T. ) ;
#15593=CARTESIAN_POINT ( 'NONE',  ( -40.00000000000000000, 100.0000000000000000, -150.2000000000005571 ) ) ;
#15594=FACE_BOUND ( 'NONE', #5426, .T. ) ;
#15601=FACE_OUTER_BOUND ( 'NONE', #4960, .T. ) ;
#15602=DIRECTION ( 'NONE',  ( -1.000000000000000000, -0.000000000000000000, -0.000000000000000000 ) ) ;
#15608=ADVANCED_FACE ( 'NONE', ( #19944 ), #1469, .F. ) ;
#15616=CARTESIAN_POINT ( 'NONE',  ( -280.8708543776413080, 269.1333820183295416, 146.7350371479513171 ) ) ;
#15617=DIRECTION ( 'NONE',  ( 0.000000000000000000, -1.000000000000000000, 0.000000000000000000 ) ) ;
#15619=CARTESIAN_POINT ( 'NONE',  ( -281.4928932188134922, -127.0000000000000568, -150.2000000000013245 ) ) ;
#15635=CARTESIAN_POINT ( 'NONE',  ( -281.1079617568159961, 269.7223300543793698, -145.4976310729377929 ) ) ;
#15637=ADVANCED_FACE ( 'NONE', ( #17904 ), #10785, .F. ) ;
#15638=EDGE_CURVE ( 'NONE', #733, #12117, #20291, .T. ) ;
#15651=DIRECTION ( 'NONE',  ( -0.000000000000000000, -0.000000000000000000, -1.000000000000000000 ) ) ;
#15657=CARTESIAN_POINT ( 'NONE',  ( 280.7095819834010513, 269.8873946496626672, 145.3113419039144958 ) ) ;
#15660=CARTESIAN_POINT ( 'NONE',  ( 45.00000000000000000, 269.9999999999999432, 0.000000000000000000 ) ) ;
#15672=DIRECTION ( 'NONE',  ( -0.000000000000000000, 0.000000000000000000, -1.000000000000000000 ) ) ;
#15683=DIRECTION ( 'NONE',  ( -1.000000000000000000, 0.000000000000000000, 0.000000000000000000 ) ) ;
#15689=CARTESIAN_POINT ( 'NONE',  ( -284.5132312761074331, 270.4054396500289954, 145.9953931959807676 ) ) ;
#15692=CARTESIAN_POINT ( 'NONE',  ( -280.4357337430841426, 269.7771650631953548, -145.9755899421581944 ) ) ;
#15700=DIRECTION ( 'NONE',  ( -0.000000000000000000, -1.000000000000000000, -1.110223024625156540E-16 ) ) ;
#15710=LINE ( 'NONE', #6642, #3438 ) ;
#15714=EDGE_CURVE ( 'NONE', #12957, #640, #10387, .T. ) ;
#15718=DIRECTION ( 'NONE',  ( -1.000000000000000000, -0.000000000000000000, -0.000000000000000000 ) ) ;
#15722=DIRECTION ( 'NONE',  ( -0.000000000000000000, 1.000000000000000000, 0.000000000000000000 ) ) ;
#15724=DIRECTION ( 'NONE',  ( 1.000000000000000000, -0.000000000000000000, -0.000000000000000000 ) ) ;
#15726=ORIENTED_EDGE ( 'NONE', *, *, #8894, .T. ) ;
#15727=CARTESIAN_POINT ( 'NONE',  ( -281.2440776823446527, 269.1610889986682196, 150.0646579186752376 ) ) ;
#15731=LINE ( 'NONE', #10181, #9259 ) ;
#15732=VECTOR ( 'NONE', #14663, 1000.000000000000000 ) ;
#15733=CARTESIAN_POINT ( 'NONE',  ( -280.4986342070537262, 269.7080393212556260, 146.1045205713626274 ) ) ;
#15747=CARTESIAN_POINT ( 'NONE',  ( -280.0000000000000568, 269.9999999999999432, -144.9999999999999716 ) ) ;
#15754=DIRECTION ( 'NONE',  ( 1.000000000000000000, 0.000000000000000000, -0.000000000000000000 ) ) ;
#15771=CARTESIAN_POINT ( 'NONE',  ( 281.6578961534456766, 269.2533442688712171, 145.8089314698393366 ) ) ;
#15796=ORIENTED_EDGE ( 'NONE', *, *, #18749, .F. ) ;
#15801=DIRECTION ( 'NONE',  ( 1.000000000000000000, -3.495664435217746987E-15, -0.000000000000000000 ) ) ;
#15810=ORIENTED_EDGE ( 'NONE', *, *, #9449, .F. ) ;
#15815=CARTESIAN_POINT ( 'NONE',  ( 280.4974534559949007, 269.7094021484633117, 146.1021437883072167 ) ) ;
#15831=ORIENTED_EDGE ( 'NONE', *, *, #8579, .T. ) ;
#15836=DIRECTION ( 'NONE',  ( 0.000000000000000000, 1.000000000000000000, 0.000000000000000000 ) ) ;
#15843=CARTESIAN_POINT ( 'NONE',  ( -280.8700598572183935, 270.9755088701073191, -149.1320353020573464 ) ) ;
#15849=EDGE_LOOP ( 'NONE', ( #5029, #9280, #5829, #12243 ) ) ;
#15854=CARTESIAN_POINT ( 'NONE',  ( -40.00000000000000000, 100.0000000000000000, 150.2000000000009550 ) ) ;
#15861=CARTESIAN_POINT ( 'NONE',  ( -281.3684637452626589, 268.4807971656550194, 150.1999999999999886 ) ) ;
#15866=FACE_OUTER_BOUND ( 'NONE', #23264, .T. ) ;
#15867=LINE ( 'NONE', #12509, #20767 ) ;
#15875=PLANE ( 'NONE',  #10447 ) ;
#15880=CARTESIAN_POINT ( 'NONE',  ( -281.7592670532760053, 269.1520027839447948, -145.8708543776411659 ) ) ;
#15900=DIRECTION ( 'NONE',  ( 0.000000000000000000, -3.495664435217746987E-15, -1.000000000000000000 ) ) ;
#15902=CARTESIAN_POINT ( 'NONE',  ( -281.4928932188134354, -127.0000000000000568, -147.2000000000012960 ) ) ;
#15904=ORIENTED_EDGE ( 'NONE', *, *, #8437, .T. ) ;
#15921=CARTESIAN_POINT ( 'NONE',  ( 281.4928932188133217, -127.0000000000000568, 152.4000000000014268 ) ) ;
#15928=CARTESIAN_POINT ( 'NONE',  ( -281.4301275412298651, 267.9452901038201844, -147.1999999999999602 ) ) ;
#15934=DIRECTION ( 'NONE',  ( 0.000000000000000000, 0.000000000000000000, 1.000000000000000000 ) ) ;
#15937=ORIENTED_EDGE ( 'NONE', *, *, #17298, .T. ) ;
#15945=VERTEX_POINT ( 'NONE', #4424 ) ;
#15960=CARTESIAN_POINT ( 'NONE',  ( 312.2000000000013529, -129.2000000000000455, -146.4928932188134070 ) ) ;
#15973=CARTESIAN_POINT ( 'NONE',  ( -280.8716261326570702, 269.1405375976307823, 146.7502846751313257 ) ) ;
#15985=DIRECTION ( 'NONE',  ( 1.000000000000000000, 0.000000000000000000, -0.000000000000000000 ) ) ;
#15992=VERTEX_POINT ( 'NONE', #20856 ) ;
#16000=DIRECTION ( 'NONE',  ( 0.000000000000000000, 0.000000000000000000, 1.000000000000000000 ) ) ;
#16007=EDGE_CURVE ( 'NONE', #6854, #3355, #17004, .T. ) ;
#16010=DIRECTION ( 'NONE',  ( 0.000000000000000000, 0.000000000000000000, 1.000000000000000000 ) ) ;
#16012=ORIENTED_EDGE ( 'NONE', *, *, #17099, .T. ) ;
#16022=CARTESIAN_POINT ( 'NONE',  ( -280.6807971656551217, 272.9999999999999432, 145.1244294735509470 ) ) ;
#16025=CARTESIAN_POINT ( 'NONE',  ( -283.1755088701073646, 271.9320353020571588, -145.6228333615949566 ) ) ;
#16026=ORIENTED_EDGE ( 'NONE', *, *, #23530, .F. ) ;
#16036=PLANE ( 'NONE',  #11986 ) ;
#16043=ORIENTED_EDGE ( 'NONE', *, *, #4415, .F. ) ;
#16047=ORIENTED_EDGE ( 'NONE', *, *, #3515, .T. ) ;
#16062=VERTEX_POINT ( 'NONE', #13654 ) ;
#16067=CARTESIAN_POINT ( 'NONE',  ( -280.7154581756739162, 271.5968359015654983, -148.5570580646226801 ) ) ;
#16069=CARTESIAN_POINT ( 'NONE',  ( -34.75000000000005684, 100.0000000000000000, 147.2000000000005855 ) ) ;
#16073=DIRECTION ( 'NONE',  ( -1.000000000000000000, 3.495664435217746987E-15, 0.000000000000000000 ) ) ;
#16074=EDGE_CURVE ( 'NONE', #20963, #14990, #11343, .T. ) ;
#16076=EDGE_LOOP ( 'NONE', ( #22478, #8481, #21952, #618, #17634, #4655, #101, #22713 ) ) ;
#16083=VERTEX_POINT ( 'NONE', #18653 ) ;
#16100=DIRECTION ( 'NONE',  ( -1.000000000000000000, -0.000000000000000000, -0.000000000000000000 ) ) ;
#16102=DIRECTION ( 'NONE',  ( 1.000000000000000000, -3.495664435217746987E-15, -0.000000000000000000 ) ) ;
#16107=EDGE_CURVE ( 'NONE', #16906, #12117, #12706, .T. ) ;
#16110=VECTOR ( 'NONE', #22497, 1000.000000000000000 ) ;
#16114=ORIENTED_EDGE ( 'NONE', *, *, #17271, .F. ) ;
#16117=PLANE ( 'NONE',  #7949 ) ;
#16119=CARTESIAN_POINT ( 'NONE',  ( -281.2439791848365758, 269.1488036478619961, 150.0335297745772039 ) ) ;
#16124=CARTESIAN_POINT ( 'NONE',  ( -288.2000000000006708, 90.00000000000102318, -35.00000000000001421 ) ) ;
#16133=LINE ( 'NONE', #19377, #9613 ) ;
#16138=PLANE ( 'NONE',  #21839 ) ;
#16141=EDGE_LOOP ( 'NONE', ( #16584, #478, #15276, #15133 ) ) ;
#16144=CARTESIAN_POINT ( 'NONE',  ( 281.4928932188133217, -127.0000000000000568, 152.4000000000014268 ) ) ;
#16146=VECTOR ( 'NONE', #14411, 1000.000000000000000 ) ;
#16151=DIRECTION ( 'NONE',  ( -0.000000000000000000, -0.000000000000000000, 1.000000000000000000 ) ) ;
#16159=ORIENTED_EDGE ( 'NONE', *, *, #21263, .F. ) ;
#16168=CIRCLE ( 'NONE', #23473, 5.199999999999982414 ) ;
#16174=AXIS2_PLACEMENT_3D ( 'NONE', #17893, #17787, #1347 ) ;
#16182=CARTESIAN_POINT ( 'NONE',  ( -45.24999999999996447, 100.0000000000000000, 150.2000000000009550 ) ) ;
#16191=AXIS2_PLACEMENT_3D ( 'NONE', #16738, #20579, #14940 ) ;
#16196=AXIS2_PLACEMENT_3D ( 'NONE', #10998, #16871, #16519 ) ;
#16216=LINE ( 'NONE', #16324, #10053 ) ;
#16217=CARTESIAN_POINT ( 'NONE',  ( -280.4357197208658476, 269.7771302778488689, 145.9755403010747159 ) ) ;
#16221=CARTESIAN_POINT ( 'NONE',  ( 40.00000000000000000, 100.0000000000000000, 150.2000000000009550 ) ) ;
#16226=COLOUR_RGB ( '',0.8941176470588234615, 0.8941176470588234615, 0.8941176470588234615 ) ;
#16245=ORIENTED_EDGE ( 'NONE', *, *, #9180, .F. ) ;
#16256=VERTEX_POINT ( 'NONE', #21212 ) ;
#16264=CARTESIAN_POINT ( 'NONE',  ( -285.0938770989753834, 269.1689414351989740, 146.2440776823445105 ) ) ;
#16295=DIRECTION ( 'NONE',  ( -0.000000000000000000, -0.000000000000000000, 1.000000000000000000 ) ) ;
#16305=CARTESIAN_POINT ( 'NONE',  ( 285.1999999999999318, 268.4807971656551331, -146.3684637452624315 ) ) ;
#16312=EDGE_CURVE ( 'NONE', #22518, #1647, #5258, .T. ) ;
#16324=CARTESIAN_POINT ( 'NONE',  ( -288.2000000000006708, 90.00000000000102318, -37.64999999999999147 ) ) ;
#16333=EDGE_LOOP ( 'NONE', ( #4463, #4622 ) ) ;
#16346=ORIENTED_EDGE ( 'NONE', *, *, #4696, .F. ) ;
#16361=DIRECTION ( 'NONE',  ( 1.000000000000000000, -0.000000000000000000, -0.000000000000000000 ) ) ;
#16365=DIRECTION ( 'NONE',  ( 0.000000000000000000, 0.000000000000000000, 1.000000000000000000 ) ) ;
#16368=CARTESIAN_POINT ( 'NONE',  ( -282.2000000000010687, -19.99999999999898392, 105.0000000000000000 ) ) ;
#16371=DIRECTION ( 'NONE',  ( 0.000000000000000000, 0.000000000000000000, 1.000000000000000000 ) ) ;
#16372=CARTESIAN_POINT ( 'NONE',  ( 280.6846668451111668, 271.7159870726002850, -148.4379565153279259 ) ) ;
#16373=VECTOR ( 'NONE', #18777, 1000.000000000000000 ) ;
#16397=ORIENTED_EDGE ( 'NONE', *, *, #9505, .T. ) ;
#16398=CARTESIAN_POINT ( 'NONE',  ( 280.1244266708878285, 269.9999999999999432, 145.2880230824754904 ) ) ;
#16407=ORIENTED_EDGE ( 'NONE', *, *, #17298, .F. ) ;
#16415=CARTESIAN_POINT ( 'NONE',  ( 285.0938770989752697, 269.1689414351989740, -146.2440776823444537 ) ) ;
#16420=ORIENTED_EDGE ( 'NONE', *, *, #16533, .T. ) ;
#16430=EDGE_CURVE ( 'NONE', #8654, #14664, #15285, .T. ) ;
#16431=VECTOR ( 'NONE', #18874, 1000.000000000000000 ) ;
#16451=DIRECTION ( 'NONE',  ( -0.000000000000000000, -0.000000000000000000, 1.000000000000000000 ) ) ;
#16452=DIRECTION ( 'NONE',  ( 1.000000000000000000, 0.000000000000000000, 0.000000000000000000 ) ) ;
#16459=ORIENTED_EDGE ( 'NONE', *, *, #14055, .T. ) ;
#16473=ORIENTED_EDGE ( 'NONE', *, *, #23317, .F. ) ;
#16474=FACE_OUTER_BOUND ( 'NONE', #17210, .T. ) ;
#16476=VECTOR ( 'NONE', #7901, 1000.000000000000000 ) ;
#16479=CARTESIAN_POINT ( 'NONE',  ( -285.2000000000000455, 267.7999999999999545, 146.4928932188134354 ) ) ;
#16485=EDGE_CURVE ( 'NONE', #8982, #22322, #22386, .T. ) ;
#16490=CIRCLE ( 'NONE', #3752, 5.249999999999991118 ) ;
#16492=CARTESIAN_POINT ( 'NONE',  ( -281.4928932188135491, 5.173457871231061435E-13, 150.2000000000009550 ) ) ;
#16494=CARTESIAN_POINT ( 'NONE',  ( -282.2000000000013529, -89.99999999999897682, 24.33333333333333215 ) ) ;
#16507=CARTESIAN_POINT ( 'NONE',  ( -280.0000000000000568, 267.7999999999999545, -146.4928932188134354 ) ) ;
#16511=CARTESIAN_POINT ( 'NONE',  ( 280.9952621458755289, 268.9079617568158938, 146.9223300543793584 ) ) ;
#16513=ORIENTED_EDGE ( 'NONE', *, *, #12377, .T. ) ;
#16519=DIRECTION ( 'NONE',  ( 0.000000000000000000, 1.000000000000000000, -4.183096374613631247E-18 ) ) ;
#16527=DIRECTION ( 'NONE',  ( 1.000000000000000000, -3.495664435217746987E-15, -0.000000000000000000 ) ) ;
#16533=EDGE_CURVE ( 'NONE', #21142, #20571, #1979, .T. ) ;
#16538=VECTOR ( 'NONE', #1289, 1000.000000000000000 ) ;
#16541=ADVANCED_FACE ( 'NONE', ( #8021 ), #8634, .F. ) ;
#16576=CIRCLE ( 'NONE', #6157, 2.649999999999971934 ) ;
#16578=CARTESIAN_POINT ( 'NONE',  ( 281.3684637452625452, 268.4807971656550762, -150.1999999999999318 ) ) ;
#16584=ORIENTED_EDGE ( 'NONE', *, *, #23556, .F. ) ;
#16592=ORIENTED_EDGE ( 'NONE', *, *, #3534, .T. ) ;
#16595=EDGE_LOOP ( 'NONE', ( #8032, #5528, #8589, #14936 ) ) ;
#16605=CARTESIAN_POINT ( 'NONE',  ( -45.00000000000000000, 272.9999999999999432, -5.249999999999991118 ) ) ;
#16620=CARTESIAN_POINT ( 'NONE',  ( 281.4928932188134354, 267.8000000000000114, -150.1999999999999318 ) ) ;
#16627=CARTESIAN_POINT ( 'NONE',  ( -282.2000000000012960, -74.99999999999899103, -90.00000000000000000 ) ) ;
#16638=ORIENTED_EDGE ( 'NONE', *, *, #11288, .F. ) ;
#16641=LINE ( 'NONE', #3812, #7734 ) ;
#16643=CARTESIAN_POINT ( 'NONE',  ( 281.9771302778490281, 268.7755403010747841, -146.0571734979477014 ) ) ;
#16650=CARTESIAN_POINT ( 'NONE',  ( 281.4928932188133217, -129.2000000000000455, 177.2000000000014097 ) ) ;
#16661=EDGE_CURVE ( 'NONE', #18758, #5006, #19946, .T. ) ;
#16669=EDGE_CURVE ( 'NONE', #9425, #12339, #22001, .T. ) ;
#16680=CARTESIAN_POINT ( 'NONE',  ( -280.5724317483737309, 269.9290760626066117, -145.2497115627124060 ) ) ;
#16682=DIRECTION ( 'NONE',  ( 0.000000000000000000, -0.000000000000000000, 1.000000000000000000 ) ) ;
#16685=DIRECTION ( 'NONE',  ( 1.000000000000000000, 0.000000000000000000, 0.000000000000000000 ) ) ;
#16692=CARTESIAN_POINT ( 'NONE',  ( 281.4928932188134354, 267.8000000000000114, -147.1999999999999318 ) ) ;
#16694=CARTESIAN_POINT ( 'NONE',  ( -100.0000000000000853, -127.0000000000000568, 152.4000000000014268 ) ) ;
#16697=CARTESIAN_POINT ( 'NONE',  ( 284.5132312761075468, 270.4054396500289954, -145.9953931959807676 ) ) ;
#16698=ADVANCED_FACE ( 'NONE', ( #20176 ), #3627, .F. ) ;
#16703=ORIENTED_EDGE ( 'NONE', *, *, #8122, .T. ) ;
#16709=EDGE_CURVE ( 'NONE', #6984, #21880, #23764, .T. ) ;
#16716=ORIENTED_EDGE ( 'NONE', *, *, #19678, .F. ) ;
#16723=CARTESIAN_POINT ( 'NONE',  ( -282.6339272673398000, 272.3699028110927429, -145.4976310729377929 ) ) ;
#16727=VERTEX_POINT ( 'NONE', #18026 ) ;
#16738=CARTESIAN_POINT ( 'NONE',  ( -282.2000000000012960, -74.99999999999899103, -90.00000000000000000 ) ) ;
#16740=DIRECTION ( 'NONE',  ( 0.000000000000000000, -1.000000000000000000, 0.000000000000000000 ) ) ;
#16744=CARTESIAN_POINT ( 'NONE',  ( 0.000000000000000000, 5.068713431065766803E-13, 147.2000000000009550 ) ) ;
#16750=VECTOR ( 'NONE', #11134, 1000.000000000000000 ) ;
#16753=FACE_OUTER_BOUND ( 'NONE', #11394, .T. ) ;
#16757=CARTESIAN_POINT ( 'NONE',  ( 280.0627246244600883, 272.9999999999999432, 145.3431883566701117 ) ) ;
#16759=CIRCLE ( 'NONE', #22694, 2.649999999999971934 ) ;
#16762=CARTESIAN_POINT ( 'NONE',  ( 281.3610889986682082, 272.8646579186752774, -145.2488155364688680 ) ) ;
#16764=CYLINDRICAL_SURFACE ( 'NONE', #19290, 5.199999999999982414 ) ;
#16767=FACE_OUTER_BOUND ( 'NONE', #10070, .T. ) ;
#16778=DIRECTION ( 'NONE',  ( 0.000000000000000000, 0.000000000000000000, 1.000000000000000000 ) ) ;
#16780=DIRECTION ( 'NONE',  ( 0.000000000000000000, -1.000000000000000000, 0.000000000000000000 ) ) ;
#16790=EDGE_CURVE ( 'NONE', #4025, #15178, #14166, .T. ) ;
#16806=LINE ( 'NONE', #5577, #9913 ) ;
#16817=ORIENTED_EDGE ( 'NONE', *, *, #13498, .F. ) ;
#16818=CARTESIAN_POINT ( 'NONE',  ( -280.3120962995436685, 272.7324007871374079, 146.6810649015077388 ) ) ;
#16825=VECTOR ( 'NONE', #16964, 1000.000000000000000 ) ;
#16832=LINE ( 'NONE', #11428, #20049 ) ;
#16834=EDGE_CURVE ( 'NONE', #10471, #10559, #16806, .T. ) ;
#16836=CARTESIAN_POINT ( 'NONE',  ( -282.2000000000000455, 269.9999999999999432, -146.4928932188134070 ) ) ;
#16848=DIRECTION ( 'NONE',  ( -0.000000000000000000, -1.000000000000000000, -0.000000000000000000 ) ) ;
#16858=CIRCLE ( 'NONE', #13814, 5.249999999999973355 ) ;
#16861=ORIENTED_EDGE ( 'NONE', *, *, #12038, .F. ) ;
#16871=DIRECTION ( 'NONE',  ( 0.000000000000000000, -4.183096374613631247E-18, -1.000000000000000000 ) ) ;
#16874=FACE_OUTER_BOUND ( 'NONE', #21649, .T. ) ;
#16883=CARTESIAN_POINT ( 'NONE',  ( -285.2000000000013529, -89.99999999999897682, 21.68333333333335844 ) ) ;
#16886=EDGE_LOOP ( 'NONE', ( #17595, #22504, #1778, #9851 ) ) ;
#16905=VERTEX_POINT ( 'NONE', #8231 ) ;
#16906=VERTEX_POINT ( 'NONE', #8343 ) ;
#16916=AXIS2_PLACEMENT_3D ( 'NONE', #16221, #10304, #3268 ) ;
#16918=ORIENTED_EDGE ( 'NONE', *, *, #2680, .F. ) ;
#16922=ADVANCED_FACE ( 'NONE', ( #8471 ), #14049, .F. ) ;
#16925=ADVANCED_FACE ( 'NONE', ( #6653 ), #17773, .F. ) ;
#16927=CARTESIAN_POINT ( 'NONE',  ( 280.9952621458755857, 270.4188186979286570, -149.5436892194421148 ) ) ;
#16934=ORIENTED_EDGE ( 'NONE', *, *, #14030, .F. ) ;
#16941=EDGE_CURVE ( 'NONE', #13423, #8654, #18364, .T. ) ;
#16942=AXIS2_PLACEMENT_3D ( 'NONE', #10723, #17945, #12089 ) ;
#16953=CARTESIAN_POINT ( 'NONE',  ( -281.4928932188134354, 267.7999999999999545, -147.1696999999999207 ) ) ;
#16962=CARTESIAN_POINT ( 'NONE',  ( 282.1696999999999775, 267.7999999999999545, 146.4928932188134922 ) ) ;
#16964=DIRECTION ( 'NONE',  ( -0.000000000000000000, -0.000000000000000000, 1.000000000000000000 ) ) ;
#16966=ORIENTED_EDGE ( 'NONE', *, *, #21945, .F. ) ;
#16982=DIRECTION ( 'NONE',  ( -1.000000000000000000, 3.495664435217746592E-15, 0.000000000000000000 ) ) ;
#16987=AXIS2_PLACEMENT_3D ( 'NONE', #14189, #22966, #10313 ) ;
#16991=CARTESIAN_POINT ( 'NONE',  ( 287.4000000000013415, -132.2000000000000455, -146.4928932188134070 ) ) ;
#16999=EDGE_LOOP ( 'NONE', ( #9702, #18505 ) ) ;
#17003=DIRECTION ( 'NONE',  ( 0.000000000000000000, 0.000000000000000000, 1.000000000000000000 ) ) ;
#17004=LINE ( 'NONE', #2489, #11531 ) ;
#17005=CARTESIAN_POINT ( 'NONE',  ( 281.9080393212556146, 268.9045205713627524, -145.9942590117596524 ) ) ;
#17010=EDGE_CURVE ( 'NONE', #3355, #3965, #8957, .T. ) ;
#17015=CARTESIAN_POINT ( 'NONE',  ( -288.2000000000010687, -19.99999999999898392, 107.6499999999999631 ) ) ;
#17019=CARTESIAN_POINT ( 'NONE',  ( 281.3520027839447835, 269.5592670532759030, -145.6220388411722126 ) ) ;
#17021=EDGE_CURVE ( 'NONE', #22116, #18256, #19688, .T. ) ;
#17024=PLANE ( 'NONE',  #15164 ) ;
#17025=VERTEX_POINT ( 'NONE', #12727 ) ;
#17035=CARTESIAN_POINT ( 'NONE',  ( -281.4928932188134922, 269.9999999999999432, -147.1999999999999318 ) ) ;
#17043=CARTESIAN_POINT ( 'NONE',  ( -281.6578961534457335, 269.2533442688712171, -145.8089314698393082 ) ) ;
#17046=CARTESIAN_POINT ( 'NONE',  ( -45.24999999999994316, 100.0000000000000000, 150.2000000000009550 ) ) ;
#17053=CARTESIAN_POINT ( 'NONE',  ( 281.2440776823445390, 268.3679143846943589, -147.1132285165672045 ) ) ;
#17054=ORIENTED_EDGE ( 'NONE', *, *, #5933, .F. ) ;
#17057=B_SPLINE_CURVE_WITH_KNOTS ( 'NONE', 3,
 ( #5813, #5913, #11384, #13324, #18697, #2158, #382, #15124, #20636, #10534, #16067, #19419, #15843, #21486, #23414, #21365, #17763, #5077, #2650, #4950 ),
 .UNSPECIFIED., .F., .F.,
 ( 4, 2, 2, 2, 2, 2, 2, 2, 2, 4 ),
 ( 2.775557561562891043E-17, 0.001035985217005784553, 0.002071970434011541351, 0.003107955651017298149, 0.003625948259520210808, 0.004143940868023123468, 0.005179926085028860316, 0.006215911302034597165, 0.007251896519040333146, 0.008287881736046069994 ),
 .UNSPECIFIED. ) ;
#17060=CARTESIAN_POINT ( 'NONE',  ( -282.2000000000012960, -74.99999999999899103, 90.00000000000000000 ) ) ;
#17065=CARTESIAN_POINT ( 'NONE',  ( 45.00000000000000000, 272.9999999999999432, -5.249999999999973355 ) ) ;
#17071=CARTESIAN_POINT ( 'NONE',  ( -281.9080393212558420, 268.9045205713626956, 145.9942590117597376 ) ) ;
#17073=VERTEX_POINT ( 'NONE', #15960 ) ;
#17074=ORIENTED_EDGE ( 'NONE', *, *, #21580, .F. ) ;
#17079=CARTESIAN_POINT ( 'NONE',  ( -285.2300000000000182, 268.4847249064868606, -146.3684637172358691 ) ) ;
#17080=EDGE_LOOP ( 'NONE', ( #6161, #23221, #21753, #1772 ) ) ;
#17082=LINE ( 'NONE', #2210, #16110 ) ;
#17089=LINE ( 'NONE', #4654, #8324 ) ;
#17091=DIRECTION ( 'NONE',  ( -1.000000000000000000, -0.000000000000000000, -0.000000000000000000 ) ) ;
#17094=LINE ( 'NONE', #15301, #11922 ) ;
#17099=EDGE_CURVE ( 'NONE', #22918, #21062, #5087, .T. ) ;
#17110=ORIENTED_EDGE ( 'NONE', *, *, #6803, .F. ) ;
#17111=DIRECTION ( 'NONE',  ( -1.000000000000000000, 0.000000000000000000, 0.000000000000000000 ) ) ;
#17115=CIRCLE ( 'NONE', #15582, 2.199999999999979750 ) ;
#17121=DIRECTION ( 'NONE',  ( 1.000000000000000000, 0.000000000000000000, 0.000000000000000000 ) ) ;
#17126=CARTESIAN_POINT ( 'NONE',  ( 279.9999999999999432, 269.9999999999999432, -144.9999999999999716 ) ) ;
#17130=VECTOR ( 'NONE', #3454, 1000.000000000000000 ) ;
#17132=ORIENTED_EDGE ( 'NONE', *, *, #21274, .T. ) ;
#17137=ADVANCED_FACE ( 'NONE', ( #2029 ), #3957, .F. ) ;
#17144=DIRECTION ( 'NONE',  ( 0.000000000000000000, -1.000000000000000000, 0.000000000000000000 ) ) ;
#17153=VECTOR ( 'NONE', #6414, 1000.000000000000000 ) ;
#17157=CARTESIAN_POINT ( 'NONE',  ( 283.9107452280323969, 271.2314821058791949, 145.8083875057489820 ) ) ;
#17159=DIRECTION ( 'NONE',  ( -0.000000000000000000, -0.000000000000000000, 1.000000000000000000 ) ) ;
#17178=CARTESIAN_POINT ( 'NONE',  ( -280.1244294735510607, 272.9999999999999432, 145.6807971656551501 ) ) ;
#17182=FACE_BOUND ( 'NONE', #12424, .T. ) ;
#17190=CARTESIAN_POINT ( 'NONE',  ( -280.2488155364688964, 272.8938770989752811, -146.3689414351990479 ) ) ;
#17199=CARTESIAN_POINT ( 'NONE',  ( 280.5758453455903805, 269.9427398886703031, 145.2488155364688964 ) ) ;
#17208=VERTEX_POINT ( 'NONE', #13080 ) ;
#17210=EDGE_LOOP ( 'NONE', ( #4108, #147, #20634, #10397 ) ) ;
#17218=CARTESIAN_POINT ( 'NONE',  ( -45.00000000000000000, 272.9999999999999432, 0.000000000000000000 ) ) ;
#17221=CARTESIAN_POINT ( 'NONE',  ( -285.2000000000007276, 75.00000000000098055, 90.00000000000000000 ) ) ;
#17228=ORIENTED_EDGE ( 'NONE', *, *, #8453, .F. ) ;
#17231=ORIENTED_EDGE ( 'NONE', *, *, #11895, .T. ) ;
#17237=ORIENTED_EDGE ( 'NONE', *, *, #23275, .F. ) ;
#17243=CARTESIAN_POINT ( 'NONE',  ( 280.6222583006965010, 271.9268706878667103, 148.1682701916307110 ) ) ;
#17244=DIRECTION ( 'NONE',  ( 6.640089860198304064E-16, 1.000000000000000000, -3.495664435217746987E-15 ) ) ;
#17259=DIRECTION ( 'NONE',  ( 0.000000000000000000, 0.000000000000000000, 1.000000000000000000 ) ) ;
#17260=VECTOR ( 'NONE', #22160, 1000.000000000000000 ) ;
#17266=EDGE_CURVE ( 'NONE', #67, #5337, #5668, .T. ) ;
#17271=EDGE_CURVE ( 'NONE', #12385, #14070, #5670, .T. ) ;
#17272=DIRECTION ( 'NONE',  ( 0.000000000000000000, 0.000000000000000000, 1.000000000000000000 ) ) ;
#17274=ORIENTED_EDGE ( 'NONE', *, *, #9514, .F. ) ;
#17289=EDGE_LOOP ( 'NONE', ( #6082, #6448, #8163, #22903 ) ) ;
#17298=EDGE_CURVE ( 'NONE', #12111, #8982, #8211, .T. ) ;
#17300=CARTESIAN_POINT ( 'NONE',  ( -280.6220388411723548, 271.9822575857424454, 148.2140793454688037 ) ) ;
#17308=CARTESIAN_POINT ( 'NONE',  ( 287.4000000000013415, -127.0000000000000568, 146.4928932188134638 ) ) ;
#17313=CARTESIAN_POINT ( 'NONE',  ( -281.2440776823445390, 268.3758453455904487, -147.1427398886702349 ) ) ;
#17314=EDGE_CURVE ( 'NONE', #13252, #3595, #22238, .T. ) ;
#17320=DIRECTION ( 'NONE',  ( 0.000000000000000000, 0.000000000000000000, 1.000000000000000000 ) ) ;
#17324=CARTESIAN_POINT ( 'NONE',  ( 280.5679143846942907, 269.9132285165672442, 145.2488155364688964 ) ) ;
#17330=CARTESIAN_POINT ( 'NONE',  ( 279.9999999999999432, 273.0000000000000000, -144.9999999999999716 ) ) ;
#17332=DIRECTION ( 'NONE',  ( 0.000000000000000000, -1.000000000000000000, -5.286776307738891306E-15 ) ) ;
#17336=VECTOR ( 'NONE', #9573, 1000.000000000000000 ) ;
#17339=EDGE_LOOP ( 'NONE', ( #1058, #16716 ) ) ;
#17355=DIRECTION ( 'NONE',  ( 0.000000000000000000, 0.000000000000000000, 1.000000000000000000 ) ) ;
#17364=AXIS2_PLACEMENT_3D ( 'NONE', #2216, #9856, #16982 ) ;
#17380=DIRECTION ( 'NONE',  ( 0.000000000000000000, -3.495664435217746987E-15, 1.000000000000000000 ) ) ;
#17397=ORIENTED_EDGE ( 'NONE', *, *, #14078, .F. ) ;
#17400=ORIENTED_EDGE ( 'NONE', *, *, #1576, .F. ) ;
#17407=CARTESIAN_POINT ( 'NONE',  ( -288.2000000000013529, -89.99999999999896261, -37.68333333333335844 ) ) ;
#17411=EDGE_CURVE ( 'NONE', #16727, #23739, #16858, .T. ) ;
#17412=VERTEX_POINT ( 'NONE', #10393 ) ;
#17426=CARTESIAN_POINT ( 'NONE',  ( 285.1999999999999318, 267.7999999999999545, 146.4928932188134922 ) ) ;
#17451=ORIENTED_EDGE ( 'NONE', *, *, #21500, .F. ) ;
#17457=CARTESIAN_POINT ( 'NONE',  ( 281.9094021484634141, 268.9021437883071712, 145.9954397628184495 ) ) ;
#17459=CARTESIAN_POINT ( 'NONE',  ( -287.4000000000014552, -129.2000000000000455, -146.4928932188134070 ) ) ;
#17460=ORIENTED_EDGE ( 'NONE', *, *, #1765, .T. ) ;
#17461=DIRECTION ( 'NONE',  ( -1.000000000000000000, 3.495664435217746987E-15, 0.000000000000000000 ) ) ;
#17475=ORIENTED_EDGE ( 'NONE', *, *, #3655, .T. ) ;
#17484=ORIENTED_EDGE ( 'NONE', *, *, #10775, .T. ) ;
#17492=DIRECTION ( 'NONE',  ( -1.000000000000000000, 0.000000000000000000, 9.860133695827843917E-17 ) ) ;
#17519=EDGE_CURVE ( 'NONE', #23739, #21291, #19894, .T. ) ;
#17525=LINE ( 'NONE', #18855, #1674 ) ;
#17526=EDGE_CURVE ( 'NONE', #16062, #2779, #9728, .T. ) ;
#17536=VECTOR ( 'NONE', #4178, 1000.000000000000000 ) ;
#17561=B_SPLINE_CURVE_WITH_KNOTS ( 'NONE', 3,
 ( #11539, #22243, #13134, #18863, #22730, #2330, #11309, #20445, #9716, #17071, #6201, #530, #18615, #6071, #13487, #4269 ),
 .UNSPECIFIED., .F., .F.,
 ( 4, 2, 2, 2, 2, 2, 2, 4 ),
 ( 0.000000000000000000, 0.0009361184303671388424, 0.001404177645550679261, 0.001872236860734219788, 0.002340296075917760316, 0.002808355291101300843, 0.003276414506284841370, 0.003744473721468381464 ),
 .UNSPECIFIED. ) ;
#17563=LINE ( 'NONE', #1011, #1114 ) ;
#17564=LINE ( 'NONE', #23476, #23501 ) ;
#17572=ORIENTED_EDGE ( 'NONE', *, *, #1221, .T. ) ;
#17574=ORIENTED_EDGE ( 'NONE', *, *, #7211, .T. ) ;
#17585=FACE_OUTER_BOUND ( 'NONE', #18499, .T. ) ;
#17590=CARTESIAN_POINT ( 'NONE',  ( 99.99999999999987210, -132.2000000000000455, 177.2000000000014097 ) ) ;
#17594=CARTESIAN_POINT ( 'NONE',  ( -285.0327955282141943, 269.1518577254344677, 146.2434055557877741 ) ) ;
#17595=ORIENTED_EDGE ( 'NONE', *, *, #16669, .F. ) ;
#17612=VECTOR ( 'NONE', #7016, 1000.000000000000000 ) ;
#17615=ORIENTED_EDGE ( 'NONE', *, *, #872, .F. ) ;
#17634=ORIENTED_EDGE ( 'NONE', *, *, #1221, .F. ) ;
#17635=CARTESIAN_POINT ( 'NONE',  ( -280.6220388411723548, 269.5350371479512432, 146.3333820183295586 ) ) ;
#17659=LINE ( 'NONE', #990, #13915 ) ;
#17666=VECTOR ( 'NONE', #20966, 1000.000000000000000 ) ;
#17668=CARTESIAN_POINT ( 'NONE',  ( -281.4928932188134922, -132.2000000000000455, -177.2000000000013529 ) ) ;
#17678=AXIS2_PLACEMENT_3D ( 'NONE', #5269, #22151, #9135 ) ;
#17686=EDGE_CURVE ( 'NONE', #5390, #2544, #17082, .T. ) ;
#17704=VECTOR ( 'NONE', #2589, 1000.000000000000000 ) ;
#17705=CARTESIAN_POINT ( 'NONE',  ( -284.1268706878666990, 270.9682701916306087, -145.8706349181168491 ) ) ;
#17717=DIRECTION ( 'NONE',  ( -0.000000000000000000, 1.000000000000000000, -0.000000000000000000 ) ) ;
#17718=CARTESIAN_POINT ( 'NONE',  ( -280.0000000000000568, 267.7999999999999545, -147.1999999999999318 ) ) ;
#17721=DIRECTION ( 'NONE',  ( -1.000000000000000000, 0.000000000000000000, -0.000000000000000000 ) ) ;
#17730=CIRCLE ( 'NONE', #1885, 2.649999999999978595 ) ;
#17731=ORIENTED_EDGE ( 'NONE', *, *, #10824, .F. ) ;
#17758=ORIENTED_EDGE ( 'NONE', *, *, #8752, .F. ) ;
#17763=CARTESIAN_POINT ( 'NONE',  ( -281.2434055557877741, 269.1518577254345246, -150.0327955282141659 ) ) ;
#17767=LINE ( 'NONE', #8466, #20684 ) ;
#17768=VERTEX_POINT ( 'NONE', #2811 ) ;
#17773=PLANE ( 'NONE',  #23394 ) ;
#17784=PLANE ( 'NONE',  #9780 ) ;
#17787=DIRECTION ( 'NONE',  ( 0.000000000000000000, -3.495664435217746987E-15, -1.000000000000000000 ) ) ;
#17805=ORIENTED_EDGE ( 'NONE', *, *, #18455, .F. ) ;
#17810=ORIENTED_EDGE ( 'NONE', *, *, #9180, .T. ) ;
#17815=DIRECTION ( 'NONE',  ( 0.000000000000000000, -1.000000000000000000, 0.000000000000000000 ) ) ;
#17822=VERTEX_POINT ( 'NONE', #11923 ) ;
#17833=DIRECTION ( 'NONE',  ( 0.000000000000000000, 1.000000000000000000, 0.000000000000000000 ) ) ;
#17836=ORIENTED_EDGE ( 'NONE', *, *, #3809, .F. ) ;
#17837=DIRECTION ( 'NONE',  ( 0.000000000000000000, -1.000000000000000000, 0.000000000000000000 ) ) ;
#17842=EDGE_CURVE ( 'NONE', #1216, #17073, #1599, .T. ) ;
#17844=CARTESIAN_POINT ( 'NONE',  ( -283.0299054689547802, 272.0295083325148084, 145.5908103165960767 ) ) ;
#17849=CARTESIAN_POINT ( 'NONE',  ( 281.2431816561009441, 268.3724317483736854, 147.1290760626067140 ) ) ;
#17881=ORIENTED_EDGE ( 'NONE', *, *, #12442, .F. ) ;
#17882=FACE_OUTER_BOUND ( 'NONE', #10995, .T. ) ;
#17893=CARTESIAN_POINT ( 'NONE',  ( 40.00000000000000000, 100.0000000000000000, 147.2000000000005855 ) ) ;
#17895=CARTESIAN_POINT ( 'NONE',  ( -281.4928932188135491, -132.2000000000000455, 177.2000000000014097 ) ) ;
#17902=EDGE_CURVE ( 'NONE', #9425, #14489, #5310, .T. ) ;
#17903=DIRECTION ( 'NONE',  ( 0.000000000000000000, -1.000000000000000000, 0.000000000000000000 ) ) ;
#17904=FACE_OUTER_BOUND ( 'NONE', #13141, .T. ) ;
#17911=ORIENTED_EDGE ( 'NONE', *, *, #12322, .T. ) ;
#17919=DIRECTION ( 'NONE',  ( 0.000000000000000000, 0.000000000000000000, 1.000000000000000000 ) ) ;
#17931=PLANE ( 'NONE',  #14176 ) ;
#17934=DIRECTION ( 'NONE',  ( -0.000000000000000000, -0.000000000000000000, 1.000000000000000000 ) ) ;
#17942=CARTESIAN_POINT ( 'NONE',  ( -280.5679143846944044, 269.9132285165672442, 145.2488155364689248 ) ) ;
#17945=DIRECTION ( 'NONE',  ( -1.000000000000000000, -0.000000000000000000, -0.000000000000000000 ) ) ;
#17950=FACE_BOUND ( 'NONE', #22610, .T. ) ;
#17959=DIRECTION ( 'NONE',  ( -1.000000000000000000, 3.495664435217746987E-15, 0.000000000000000000 ) ) ;
#17962=AXIS2_PLACEMENT_3D ( 'NONE', #4881, #19597, #14435 ) ;
#17973=CARTESIAN_POINT ( 'NONE',  ( -287.4000000000014552, -127.0000000000000568, 146.4928932188134638 ) ) ;
#17978=EDGE_CURVE ( 'NONE', #3965, #8982, #20178, .T. ) ;
#17981=CARTESIAN_POINT ( 'NONE',  ( -288.2000000000013529, -89.99999999999896261, -42.98333333333330586 ) ) ;
#17983=ORIENTED_EDGE ( 'NONE', *, *, #10154, .F. ) ;
#17995=ORIENTED_EDGE ( 'NONE', *, *, #22344, .F. ) ;
#18003=EDGE_CURVE ( 'NONE', #6854, #11293, #1087, .T. ) ;
#18014=CARTESIAN_POINT ( 'NONE',  ( 34.75000000000005684, 100.0000000000000000, 150.2000000000009550 ) ) ;
#18026=CARTESIAN_POINT ( 'NONE',  ( -45.00000000000000000, 269.9999999999999432, 5.249999999999973355 ) ) ;
#18045=CARTESIAN_POINT ( 'NONE',  ( 285.1999999999999318, 267.7999999999999545, -146.4928932188134070 ) ) ;
#18049=PLANE ( 'NONE',  #15035 ) ;
#18050=FACE_OUTER_BOUND ( 'NONE', #9685, .T. ) ;
#18056=VECTOR ( 'NONE', #16151, 1000.000000000000000 ) ;
#18059=LINE ( 'NONE', #1507, #18866 ) ;
#18061=CARTESIAN_POINT ( 'NONE',  ( -283.1956429438696432, 271.9582675804705332, 145.6220388411722695 ) ) ;
#18075=LINE ( 'NONE', #1530, #21493 ) ;
#18084=ORIENTED_EDGE ( 'NONE', *, *, #19441, .T. ) ;
#18087=CARTESIAN_POINT ( 'NONE',  ( -281.4928932188135491, -127.0000000000000568, 150.2000000000013813 ) ) ;
#18089=B_SPLINE_SURFACE_WITH_KNOTS ( 'NONE', 1, 3, ( 
 ( #9942, #22833, #858, #11776, #4615, #17300, #2554, #21275, #8238, #19328 ),
 ( #6300, #15861, #15727, #13711, #21030, #8350, #749, #8133, #17178, #6547 ),
 ( #6418, #4491, #971, #12138, #2788, #4253, #15504, #4368, #23068, #2431 ),
 ( #19436, #11898, #11662, #19206, #15616, #17635, #19086, #22945, #13823, #21149 ) ),
 .UNSPECIFIED., .F., .F., .F.,
 ( 2, 1, 1, 2 ),
 ( 4, 2, 2, 2, 4 ),
 ( -0.01000000000000000021, 0.000000000000000000, 1.000000000000000000, 1.010099999999999998 ),
 ( 0.000000000000000000, 0.2500000000000000000, 0.5000000000000000000, 0.7500000000000000000, 1.000000000000000000 ),
 .UNSPECIFIED. ) ;
#18096=VERTEX_POINT ( 'NONE', #18843 ) ;
#18097=CARTESIAN_POINT ( 'NONE',  ( 280.1244294735508333, 272.9999999999999432, 145.6807971656549228 ) ) ;
#18109=CARTESIAN_POINT ( 'NONE',  ( 283.2140793454687469, 271.9822575857424454, -145.6220388411722126 ) ) ;
#18120=EDGE_LOOP ( 'NONE', ( #17805, #23286, #16407, #1537 ) ) ;
#18123=DIRECTION ( 'NONE',  ( -1.000000000000000000, -3.491481338843133355E-15, 0.000000000000000000 ) ) ;
#18128=VECTOR ( 'NONE', #4585, 1000.000000000000000 ) ;
#18135=DIRECTION ( 'NONE',  ( 0.000000000000000000, -1.000000000000000000, -4.183096374613631247E-18 ) ) ;
#18136=CARTESIAN_POINT ( 'NONE',  ( -281.3673618604588000, 268.0905802150185195, 147.2000000000000171 ) ) ;
#18139=DIRECTION ( 'NONE',  ( -1.000000000000000000, -0.000000000000000000, -0.000000000000000000 ) ) ;
#18174=FACE_OUTER_BOUND ( 'NONE', #22682, .T. ) ;
#18177=CARTESIAN_POINT ( 'NONE',  ( 280.6842353883613441, 269.4574776399289249, -146.4538215477170127 ) ) ;
#18183=CARTESIAN_POINT ( 'NONE',  ( 280.8706349181168775, 270.9682701916305518, -149.1268706878665284 ) ) ;
#18187=CYLINDRICAL_SURFACE ( 'NONE', #11442, 5.199999999999982414 ) ;
#18208=CARTESIAN_POINT ( 'NONE',  ( 281.4928932188133217, 267.7999999999999545, 147.1696999999999775 ) ) ;
#18214=DIRECTION ( 'NONE',  ( -1.000000000000000000, -0.000000000000000000, -0.000000000000000000 ) ) ;
#18215=CARTESIAN_POINT ( 'NONE',  ( 0.000000000000000000, 0.000000000000000000, -147.2000000000008981 ) ) ;
#18219=CARTESIAN_POINT ( 'NONE',  ( 40.00000000000000000, 100.0000000000000000, -147.2000000000005571 ) ) ;
#18220=VECTOR ( 'NONE', #7607, 1000.000000000000000 ) ;
#18232=ORIENTED_EDGE ( 'NONE', *, *, #12033, .F. ) ;
#18235=CARTESIAN_POINT ( 'NONE',  ( -282.2000000000006708, 90.00000000000102318, -35.00000000000001421 ) ) ;
#18239=CARTESIAN_POINT ( 'NONE',  ( 99.99999999999997158, 34.99999999999995026, -113.4834095219707848 ) ) ;
#18245=ORIENTED_EDGE ( 'NONE', *, *, #17519, .T. ) ;
#18251=CIRCLE ( 'NONE', #5935, 2.199999999999979750 ) ;
#18253=CARTESIAN_POINT ( 'NONE',  ( -282.2000000000014666, -127.0000000000000568, 146.4928932188134638 ) ) ;
#18256=VERTEX_POINT ( 'NONE', #4205 ) ;
#18260=ORIENTED_EDGE ( 'NONE', *, *, #21500, .T. ) ;
#18261=ORIENTED_EDGE ( 'NONE', *, *, #8614, .T. ) ;
#18266=CARTESIAN_POINT ( 'NONE',  ( -285.2000000000006708, 90.00000000000102318, -37.64999999999999147 ) ) ;
#18268=B_SPLINE_SURFACE_WITH_KNOTS ( 'NONE', 1, 3, ( 
 ( #9842, #2451, #15283, #5847, #13618, #15048, #13370, #13256, #7779, #20451 ),
 ( #22385, #22494, #2569, #20564, #770, #6211, #22614, #11796, #5962, #11679 ),
 ( #22249, #22743, #20681, #4138, #8152, #9724, #3905, #17199, #20928, #15401 ),
 ( #16962, #4015, #19110, #292, #11553, #11430, #5725, #17324, #4388, #13499 ) ),
 .UNSPECIFIED., .F., .F., .F.,
 ( 2, 1, 1, 2 ),
 ( 4, 2, 2, 2, 4 ),
 ( -0.01000000000000000021, 0.000000000000000000, 1.000000000000000000, 1.010099999999999998 ),
 ( 0.000000000000000000, 0.2500000000000000000, 0.5000000000000000000, 0.7500000000000000000, 1.000000000000000000 ),
 .UNSPECIFIED. ) ;
#18271=CARTESIAN_POINT ( 'NONE',  ( -287.4000000000014552, -127.0000000000000568, 146.4928932188134638 ) ) ;
#18273=ORIENTED_EDGE ( 'NONE', *, *, #16430, .F. ) ;
#18275=CARTESIAN_POINT ( 'NONE',  ( 0.000000000000000000, -132.2000000000000455, 177.2000000000014097 ) ) ;
#18276=ORIENTED_EDGE ( 'NONE', *, *, #10516, .F. ) ;
#18277=CARTESIAN_POINT ( 'NONE',  ( 280.4357197208658476, 269.7771302778488121, -145.9755403010746875 ) ) ;
#18280=CARTESIAN_POINT ( 'NONE',  ( -284.5436892194422285, 270.4188186979286002, 145.9952621458756425 ) ) ;
#18283=CARTESIAN_POINT ( 'NONE',  ( 280.1247002395579102, 272.9663407402831581, -145.6822561791009321 ) ) ;
#18284=EDGE_CURVE ( 'NONE', #16905, #9249, #20244, .T. ) ;
#18292=CYLINDRICAL_SURFACE ( 'NONE', #17678, 2.649999999999971934 ) ;
#18293=EDGE_CURVE ( 'NONE', #17025, #19104, #11365, .T. ) ;
#18296=CARTESIAN_POINT ( 'NONE',  ( 34.75000000000005684, 100.0000000000000000, -150.2000000000005571 ) ) ;
#18303=DIRECTION ( 'NONE',  ( -0.000000000000000000, 1.000000000000000000, -0.000000000000000000 ) ) ;
#18311=CARTESIAN_POINT ( 'NONE',  ( 281.2440776823444253, 268.3679143846943020, 147.1132285165672329 ) ) ;
#18322=CARTESIAN_POINT ( 'NONE',  ( -281.4928932188135491, -129.2000000000000455, 152.4000000000014268 ) ) ;
#18325=ORIENTED_EDGE ( 'NONE', *, *, #19088, .T. ) ;
#18330=ADVANCED_FACE ( 'NONE', ( #2512 ), #3952, .T. ) ;
#18357=ORIENTED_EDGE ( 'NONE', *, *, #7055, .T. ) ;
#18359=DIRECTION ( 'NONE',  ( 0.000000000000000000, 0.000000000000000000, 1.000000000000000000 ) ) ;
#18364=CIRCLE ( 'NONE', #22221, 5.249999999999949374 ) ;
#18365=CARTESIAN_POINT ( 'NONE',  ( 280.9952621458755857, 268.8927021017107108, -146.8958543268121559 ) ) ;
#18367=DIRECTION ( 'NONE',  ( 0.000000000000000000, 0.000000000000000000, 1.000000000000000000 ) ) ;
#18372=AXIS2_PLACEMENT_3D ( 'NONE', #20646, #18829, #503 ) ;
#18374=EDGE_LOOP ( 'NONE', ( #12645, #14216 ) ) ;
#18380=ADVANCED_FACE ( 'NONE', ( #689 ), #4190, .F. ) ;
#18390=ORIENTED_EDGE ( 'NONE', *, *, #21277, .F. ) ;
#18391=CARTESIAN_POINT ( 'NONE',  ( 280.8716261326570134, 269.1405375976307255, -146.7502846751312120 ) ) ;
#18410=LINE ( 'NONE', #5398, #4587 ) ;
#18424=CARTESIAN_POINT ( 'NONE',  ( 279.9999999999999432, 272.9999999999999432, 145.0000000000000284 ) ) ;
#18439=ORIENTED_EDGE ( 'NONE', *, *, #17266, .F. ) ;
#18452=VECTOR ( 'NONE', #23804, 1000.000000000000000 ) ;
#18455=EDGE_CURVE ( 'NONE', #5006, #539, #18662, .T. ) ;
#18459=DIRECTION ( 'NONE',  ( 1.000000000000000000, 0.000000000000000000, 0.000000000000000000 ) ) ;
#18460=EDGE_CURVE ( 'NONE', #14699, #17768, #10068, .T. ) ;
#18466=VERTEX_POINT ( 'NONE', #12451 ) ;
#18472=CARTESIAN_POINT ( 'NONE',  ( -285.2000000000011255, -29.99999999999898037, -107.6499999999999631 ) ) ;
#18480=CARTESIAN_POINT ( 'NONE',  ( -282.2000000000000455, 268.0905802150184627, -146.3673618604586579 ) ) ;
#18482=DIRECTION ( 'NONE',  ( -0.000000000000000000, 1.000000000000000000, 0.000000000000000000 ) ) ;
#18493=CARTESIAN_POINT ( 'NONE',  ( 280.8708543776411943, 269.1520027839448517, -146.7592670532759485 ) ) ;
#18495=VECTOR ( 'NONE', #3609, 1000.000000000000000 ) ;
#18499=EDGE_LOOP ( 'NONE', ( #7569, #8108, #22671, #16966 ) ) ;
#18503=LINE ( 'NONE', #17060, #17336 ) ;
#18505=ORIENTED_EDGE ( 'NONE', *, *, #23212, .T. ) ;
#18515=CARTESIAN_POINT ( 'NONE',  ( -45.24999999999994316, 100.0000000000000000, -150.2000000000005571 ) ) ;
#18525=CARTESIAN_POINT ( 'NONE',  ( -282.2000000000014666, -127.0000000000000568, -144.9999999999999716 ) ) ;
#18526=CARTESIAN_POINT ( 'NONE',  ( -281.4928932188134354, 267.8000000000000114, -147.1999999999999318 ) ) ;
#18527=CARTESIAN_POINT ( 'NONE',  ( -35.00000000000000711, 4.286263797015349166E-15, -150.2000000000008981 ) ) ;
#18545=CARTESIAN_POINT ( 'NONE',  ( 281.4928932188133786, -132.2000000000000455, 7.703011046602857601E-15 ) ) ;
#18547=EDGE_CURVE ( 'NONE', #21466, #640, #1359, .T. ) ;
#18553=DIRECTION ( 'NONE',  ( 1.000000000000000000, 0.000000000000000000, -0.000000000000000000 ) ) ;
#18557=ORIENTED_EDGE ( 'NONE', *, *, #4795, .F. ) ;
#18558=CARTESIAN_POINT ( 'NONE',  ( -282.2000000000008981, 30.00000000000101963, -105.0000000000000142 ) ) ;
#18563=DIRECTION ( 'NONE',  ( 0.000000000000000000, -1.000000000000000000, -5.286776307738891306E-15 ) ) ;
#18571=ORIENTED_EDGE ( 'NONE', *, *, #8816, .T. ) ;
#18572=DIRECTION ( 'NONE',  ( -1.000000000000000000, -0.000000000000000000, -0.000000000000000000 ) ) ;
#18578=ORIENTED_EDGE ( 'NONE', *, *, #7960, .T. ) ;
#18579=DIRECTION ( 'NONE',  ( 6.640089860198304064E-16, 1.000000000000000000, -3.495664435217746987E-15 ) ) ;
#18585=DIRECTION ( 'NONE',  ( -1.000000000000000000, 0.000000000000000000, 0.000000000000000000 ) ) ;
#18613=FACE_OUTER_BOUND ( 'NONE', #5136, .T. ) ;
#18615=CARTESIAN_POINT ( 'NONE',  ( -282.1290760626067708, 268.3724317483737423, 146.2431816561009725 ) ) ;
#18620=MECHANICAL_DESIGN_GEOMETRIC_PRESENTATION_REPRESENTATION('',(#12137),#7447);
#18653=CARTESIAN_POINT ( 'NONE',  ( -287.4000000000014552, -132.2000000000000455, 146.4928932188134638 ) ) ;
#18655=AXIS2_PLACEMENT_3D ( 'NONE', #3368, #20266, #18459 ) ;
#18661=ORIENTED_EDGE ( 'NONE', *, *, #12480, .T. ) ;
#18662=LINE ( 'NONE', #19031, #14120 ) ;
#18671=FACE_BOUND ( 'NONE', #8441, .T. ) ;
#18687=ORIENTED_EDGE ( 'NONE', *, *, #7973, .T. ) ;
#18696=LINE ( 'NONE', #14994, #3837 ) ;
#18697=CARTESIAN_POINT ( 'NONE',  ( -280.3118087683467365, 272.7329465209279533, -146.6795879751482801 ) ) ;
#18700=DIRECTION ( 'NONE',  ( 0.000000000000000000, -1.000000000000000000, 0.000000000000000000 ) ) ;
#18703=EDGE_CURVE ( 'NONE', #16256, #9824, #5146, .T. ) ;
#18707=FACE_BOUND ( 'NONE', #2047, .T. ) ;
#18708=DIRECTION ( 'NONE',  ( -0.000000000000000000, 0.000000000000000000, 1.000000000000000000 ) ) ;
#18710=ORIENTED_EDGE ( 'NONE', *, *, #17021, .T. ) ;
#18728=CARTESIAN_POINT ( 'NONE',  ( -280.6846668451111668, 271.7159870726003987, 148.4379565153279827 ) ) ;
#18731=DIRECTION ( 'NONE',  ( 0.000000000000000000, 0.000000000000000000, -1.000000000000000000 ) ) ;
#18733=CARTESIAN_POINT ( 'NONE',  ( -280.8708543776411943, 270.9956429438695409, -149.1582675804705218 ) ) ;
#18740=DIRECTION ( 'NONE',  ( -1.000000000000000000, 3.495664435217746592E-15, -0.000000000000000000 ) ) ;
#18742=ADVANCED_FACE ( 'NONE', ( #21690 ), #18187, .T. ) ;
#18744=CARTESIAN_POINT ( 'NONE',  ( -285.2300000000000182, 267.7999999999999545, -146.4928932188134354 ) ) ;
#18749=EDGE_CURVE ( 'NONE', #10685, #9425, #1525, .T. ) ;
#18755=PLANE ( 'NONE',  #17364 ) ;
#18758=VERTEX_POINT ( 'NONE', #12807 ) ;
#18770=CARTESIAN_POINT ( 'NONE',  ( -280.0000000000000568, 269.9999999999999432, 145.0000000000000284 ) ) ;
#18777=DIRECTION ( 'NONE',  ( -0.000000000000000000, 1.000000000000000000, -3.495664435217746987E-15 ) ) ;
#18786=CARTESIAN_POINT ( 'NONE',  ( 281.1807969192696532, 269.4810649015076933, 149.9324007871373681 ) ) ;
#18803=AXIS2_PLACEMENT_3D ( 'NONE', #20210, #3660, #7306 ) ;
#18806=CARTESIAN_POINT ( 'NONE',  ( -281.4928932188135491, 267.7999999999999545, 145.0000000000000284 ) ) ;
#18808=DIRECTION ( 'NONE',  ( 1.000000000000000000, -0.000000000000000000, -0.000000000000000000 ) ) ;
#18817=AXIS2_PLACEMENT_3D ( 'NONE', #8787, #15683, #8306 ) ;
#18822=CARTESIAN_POINT ( 'NONE',  ( -280.7095819834008807, 269.8873946496624399, -145.3113419039144105 ) ) ;
#18826=LINE ( 'NONE', #2298, #4993 ) ;
#18829=DIRECTION ( 'NONE',  ( -1.000000000000000000, -0.000000000000000000, -0.000000000000000000 ) ) ;
#18843=CARTESIAN_POINT ( 'NONE',  ( -285.2000000000013529, -89.99999999999897682, 26.98333333333330231 ) ) ;
#18845=ORIENTED_EDGE ( 'NONE', *, *, #22699, .T. ) ;
#18852=DIRECTION ( 'NONE',  ( 0.000000000000000000, 1.000000000000000000, -3.495664435217746987E-15 ) ) ;
#18855=CARTESIAN_POINT ( 'NONE',  ( 281.4928932188133217, -132.2000000000000455, 177.2000000000014097 ) ) ;
#18859=CARTESIAN_POINT ( 'NONE',  ( 281.4928932188134354, 267.8000000000000114, -144.9999999999999716 ) ) ;
#18863=CARTESIAN_POINT ( 'NONE',  ( -280.9755899421581375, 269.7771650631953548, 145.4357337430840573 ) ) ;
#18866=VECTOR ( 'NONE', #8901, 1000.000000000000000 ) ;
#18867=VECTOR ( 'NONE', #12904, 1000.000000000000000 ) ;
#18873=CARTESIAN_POINT ( 'NONE',  ( -7.690461757479017101E-15, -129.2000000000000455, 0.000000000000000000 ) ) ;
#18874=DIRECTION ( 'NONE',  ( -3.495664435217746987E-15, -1.000000000000000000, 0.000000000000000000 ) ) ;
#18878=VECTOR ( 'NONE', #12206, 1000.000000000000000 ) ;
#18880=CARTESIAN_POINT ( 'NONE',  ( 280.0627246250093094, 273.0000000000000000, -145.3431883596742011 ) ) ;
#18884=CARTESIAN_POINT ( 'NONE',  ( 99.99999999999987210, -132.2000000000003013, 177.2000000000014097 ) ) ;
#18890=CARTESIAN_POINT ( 'NONE',  ( -312.2000000000014666, -129.2000000000000455, -146.4928932188134070 ) ) ;
#18899=DIRECTION ( 'NONE',  ( 0.000000000000000000, -1.000000000000000000, 0.000000000000000000 ) ) ;
#18918=B_SPLINE_CURVE_WITH_KNOTS ( 'NONE', 3,
 ( #16620, #9369, #3441, #22141, #14455, #12666, #20325, #10858, #18183, #1627, #9008, #16372, #23720, #7175, #14567, #21905, #10961, #18283, #18880, #17330 ),
 .UNSPECIFIED., .F., .F.,
 ( 4, 2, 2, 2, 2, 2, 2, 2, 2, 4 ),
 ( 0.000000000000000000, 0.001035985217005741836, 0.002071970434011483671, 0.003107955651017225290, 0.003625948259520141419, 0.004143940868023057549, 0.005179926085028801336, 0.006215911302034544256, 0.007251896519040288043, 0.008287881736046031830 ),
 .UNSPECIFIED. ) ;
#18921=CARTESIAN_POINT ( 'NONE',  ( 280.1245861693739130, 272.9663417894421968, 145.6816199723481304 ) ) ;
#18924=EDGE_LOOP ( 'NONE', ( #8569, #13316, #477, #14462 ) ) ;
#18929=ORIENTED_EDGE ( 'NONE', *, *, #20619, .T. ) ;
#18933=CARTESIAN_POINT ( 'NONE',  ( 0.000000000000000000, -127.0000000000000568, 150.2000000000013813 ) ) ;
#18936=ORIENTED_EDGE ( 'NONE', *, *, #4596, .T. ) ;
#18937=CYLINDRICAL_SURFACE ( 'NONE', #6338, 5.199999999999982414 ) ;
#18939=ORIENTED_EDGE ( 'NONE', *, *, #12033, .T. ) ;
#18941=ORIENTED_EDGE ( 'NONE', *, *, #10549, .T. ) ;
#18949=CARTESIAN_POINT ( 'NONE',  ( 282.6054396500288703, 272.3132312761072171, 145.4975000228326678 ) ) ;
#18952=DIRECTION ( 'NONE',  ( 1.000000000000000000, 0.000000000000000000, 0.000000000000000000 ) ) ;
#18957=EDGE_CURVE ( 'NONE', #8986, #17768, #4154, .T. ) ;
#18965=CARTESIAN_POINT ( 'NONE',  ( 283.9159870726004442, 271.2379565153281078, -145.8082263737022117 ) ) ;
#18976=DIRECTION ( 'NONE',  ( -0.000000000000000000, -1.000000000000000000, -3.495664435217746987E-15 ) ) ;
#18982=ADVANCED_FACE ( 'NONE', ( #2463 ), #18755, .F. ) ;
#18984=DIRECTION ( 'NONE',  ( 0.000000000000000000, 0.000000000000000000, -1.000000000000000000 ) ) ;
#18997=CARTESIAN_POINT ( 'NONE',  ( 40.00000000000000000, 100.0000000000000000, -147.2000000000005571 ) ) ;
#19000=LINE ( 'NONE', #549, #225 ) ;
#19009=DIRECTION ( 'NONE',  ( -1.000000000000000000, -0.000000000000000000, -0.000000000000000000 ) ) ;
#19022=AXIS2_PLACEMENT_3D ( 'NONE', #21615, #5071, #12591 ) ;
#19025=ORIENTED_EDGE ( 'NONE', *, *, #17519, .F. ) ;
#19027=CARTESIAN_POINT ( 'NONE',  ( 281.4928932188133786, -127.0000000000000568, -150.2000000000013245 ) ) ;
#19028=ADVANCED_FACE ( 'NONE', ( #21306 ), #4399, .F. ) ;
#19031=CARTESIAN_POINT ( 'NONE',  ( -285.2000000000000455, 267.7999999999999545, 146.4928932188134638 ) ) ;
#19035=ORIENTED_EDGE ( 'NONE', *, *, #23777, .T. ) ;
#19036=CARTESIAN_POINT ( 'NONE',  ( -312.2000000000014666, -132.2000000000000455, -146.4928932188134070 ) ) ;
#19038=DIRECTION ( 'NONE',  ( -1.000000000000000000, 0.000000000000000000, 0.000000000000000000 ) ) ;
#19044=ORIENTED_EDGE ( 'NONE', *, *, #22574, .T. ) ;
#19052=EDGE_LOOP ( 'NONE', ( #13710, #9907, #12063, #10193 ) ) ;
#19054=DIRECTION ( 'NONE',  ( 3.700743415417189520E-15, 1.000000000000000000, 0.000000000000000000 ) ) ;
#19066=AXIS2_PLACEMENT_3D ( 'NONE', #16368, #14565, #11205 ) ;
#19070=FACE_OUTER_BOUND ( 'NONE', #21924, .T. ) ;
#19071=ORIENTED_EDGE ( 'NONE', *, *, #15638, .F. ) ;
#19079=AXIS2_PLACEMENT_3D ( 'NONE', #14746, #3598, #20151 ) ;
#19083=CARTESIAN_POINT ( 'NONE',  ( 283.4314821058791836, 271.7107452280323514, -145.6845057130644818 ) ) ;
#19084=VERTEX_POINT ( 'NONE', #22976 ) ;
#19086=CARTESIAN_POINT ( 'NONE',  ( -280.4976310729379065, 269.6958543268121957, 146.0927021017107563 ) ) ;
#19087=CYLINDRICAL_SURFACE ( 'NONE', #6522, 5.249999999999942268 ) ;
#19088=EDGE_CURVE ( 'NONE', #12339, #18758, #4757, .T. ) ;
#19097=VECTOR ( 'NONE', #13432, 1000.000000000000000 ) ;
#19104=VERTEX_POINT ( 'NONE', #1370 ) ;
#19110=CARTESIAN_POINT ( 'NONE',  ( 282.1132285165672329, 268.3679143846943020, 146.2440776823445958 ) ) ;
#19119=EDGE_CURVE ( 'NONE', #4309, #13384, #18696, .T. ) ;
#19131=LINE ( 'NONE', #10112, #1701 ) ;
#19144=CARTESIAN_POINT ( 'NONE',  ( 287.4000000000013415, -132.2000000000000455, 146.4928932188134638 ) ) ;
#19156=CARTESIAN_POINT ( 'NONE',  ( 280.2840560642350738, 269.9696999999999889, -145.1244266425809144 ) ) ;
#19165=ORIENTED_EDGE ( 'NONE', *, *, #17010, .T. ) ;
#19171=VECTOR ( 'NONE', #10512, 1000.000000000000000 ) ;
#19189=DIRECTION ( 'NONE',  ( 1.000000000000000000, 3.495664435217746987E-15, 0.000000000000000000 ) ) ;
#19206=CARTESIAN_POINT ( 'NONE',  ( -280.9952621458756994, 268.8927021017106540, 146.8958543268122128 ) ) ;
#19212=VECTOR ( 'NONE', #20867, 1000.000000000000000 ) ;
#19215=DIRECTION ( 'NONE',  ( -1.000000000000000000, -0.000000000000000000, -0.000000000000000000 ) ) ;
#19243=DIRECTION ( 'NONE',  ( 1.000000000000000000, -3.491481338843133355E-15, 0.000000000000000000 ) ) ;
#19245=LINE ( 'NONE', #13514, #21037 ) ;
#19251=AXIS2_PLACEMENT_3D ( 'NONE', #5486, #1622, #16365 ) ;
#19270=AXIS2_PLACEMENT_3D ( 'NONE', #7603, #14995, #22338 ) ;
#19277=ORIENTED_EDGE ( 'NONE', *, *, #20885, .T. ) ;
#19287=VECTOR ( 'NONE', #20481, 1000.000000000000000 ) ;
#19289=CARTESIAN_POINT ( 'NONE',  ( -280.6816199723483578, 272.9663417894423105, 145.1245861693739698 ) ) ;
#19290=AXIS2_PLACEMENT_3D ( 'NONE', #15461, #19038, #22429 ) ;
#19297=EDGE_CURVE ( 'NONE', #6984, #9249, #13582, .T. ) ;
#19301=CARTESIAN_POINT ( 'NONE',  ( -280.0000000000000568, 272.9999999999999432, 145.0000000000000284 ) ) ;
#19310=VERTEX_POINT ( 'NONE', #4222 ) ;
#19315=B_SPLINE_CURVE_WITH_KNOTS ( 'NONE', 3,
 ( #1936, #18480, #14757, #9326, #9689, #22090, #17043, #384, #11645, #5815, #11153, #18822, #16680, #2295, #497, #7746 ),
 .UNSPECIFIED., .F., .F.,
 ( 4, 2, 2, 2, 2, 2, 2, 4 ),
 ( 0.000000000000000000, 0.0009361184303672340353, 0.001404177645550768599, 0.001872236860734303489, 0.002340296075917837944, 0.002808355291101372834, 0.003276414506284907290, 0.003744473721468442179 ),
 .UNSPECIFIED. ) ;
#19328=CARTESIAN_POINT ( 'NONE',  ( -280.0000000000000568, 273.0299999999999159, 145.0000000000000284 ) ) ;
#19340=ORIENTED_EDGE ( 'NONE', *, *, #1321, .T. ) ;
#19362=ORIENTED_EDGE ( 'NONE', *, *, #8706, .T. ) ;
#19377=CARTESIAN_POINT ( 'NONE',  ( 281.4928932188134354, -132.2000000000000455, -152.4000000000013131 ) ) ;
#19383=EDGE_LOOP ( 'NONE', ( #17983, #6467, #21995, #7019 ) ) ;
#19391=EDGE_CURVE ( 'NONE', #5386, #4309, #15710, .T. ) ;
#19398=CARTESIAN_POINT ( 'NONE',  ( -280.9942590117597661, 268.9045205713627524, -146.9080393212555862 ) ) ;
#19402=VECTOR ( 'NONE', #4123, 1000.000000000000000 ) ;
#19407=ORIENTED_EDGE ( 'NONE', *, *, #16312, .F. ) ;
#19414=ORIENTED_EDGE ( 'NONE', *, *, #15523, .T. ) ;
#19419=CARTESIAN_POINT ( 'NONE',  ( -280.8082263737021549, 271.2379565153278804, -148.9159870726003874 ) ) ;
#19424=CARTESIAN_POINT ( 'NONE',  ( 281.4928932188133217, -132.2000000000000455, 177.2000000000014097 ) ) ;
#19436=CARTESIAN_POINT ( 'NONE',  ( -281.4928932188135491, 267.7999999999999545, 147.1696999999999775 ) ) ;
#19439=ADVANCED_FACE ( 'NONE', ( #7218 ), #22303, .F. ) ;
#19441=EDGE_CURVE ( 'NONE', #5160, #7573, #16576, .T. ) ;
#19452=CIRCLE ( 'NONE', #7894, 2.649999999999971934 ) ;
#19461=ORIENTED_EDGE ( 'NONE', *, *, #5471, .T. ) ;
#19466=DIRECTION ( 'NONE',  ( 0.000000000000000000, -1.000000000000000000, 0.000000000000000000 ) ) ;
#19474=ORIENTED_EDGE ( 'NONE', *, *, #10406, .T. ) ;
#19475=( NAMED_UNIT ( * ) SI_UNIT ( $, .STERADIAN. ) SOLID_ANGLE_UNIT ( ) );
#19480=CARTESIAN_POINT ( 'NONE',  ( 281.3429506979391590, 269.5484459290825043, 145.6225751257468062 ) ) ;
#19487=AXIS2_PLACEMENT_3D ( 'NONE', #9066, #14, #16780 ) ;
#19488=EDGE_CURVE ( 'NONE', #8023, #13119, #4967, .T. ) ;
#19497=ADVANCED_FACE ( 'NONE', ( #9170 ), #21350, .F. ) ;
#19505=VERTEX_POINT ( 'NONE', #20982 ) ;
#19519=CARTESIAN_POINT ( 'NONE',  ( -281.0571734979477014, 268.7755403010746136, -146.9771302778488007 ) ) ;
#19522=ORIENTED_EDGE ( 'NONE', *, *, #22580, .F. ) ;
#19525=EDGE_CURVE ( 'NONE', #10936, #3608, #6134, .T. ) ;
#19543=LINE ( 'NONE', #3138, #505 ) ;
#19551=ORIENTED_EDGE ( 'NONE', *, *, #11141, .F. ) ;
#19556=ORIENTED_EDGE ( 'NONE', *, *, #8453, .T. ) ;
#19563=FACE_BOUND ( 'NONE', #23082, .T. ) ;
#19571=ORIENTED_EDGE ( 'NONE', *, *, #14030, .T. ) ;
#19580=CIRCLE ( 'NONE', #22675, 2.649999999999971934 ) ;
#19597=DIRECTION ( 'NONE',  ( -0.000000000000000000, 1.000000000000000000, -0.000000000000000000 ) ) ;
#19610=DIRECTION ( 'NONE',  ( -0.000000000000000000, -0.000000000000000000, 1.000000000000000000 ) ) ;
#19615=CARTESIAN_POINT ( 'NONE',  ( -288.2000000000010687, -19.99999999999898392, 102.3500000000000227 ) ) ;
#19626=CIRCLE ( 'NONE', #2287, 2.649999999999971934 ) ;
#19635=LINE ( 'NONE', #5392, #17130 ) ;
#19640=DIRECTION ( 'NONE',  ( 1.000000000000000000, 9.912705577010325549E-17, 3.465149234233960866E-31 ) ) ;
#19643=PLANE ( 'NONE',  #23479 ) ;
#19650=CARTESIAN_POINT ( 'NONE',  ( 280.9942590117597092, 268.9045205713625819, 146.9080393212557567 ) ) ;
#19654=VECTOR ( 'NONE', #5677, 1000.000000000000000 ) ;
#19659=EDGE_LOOP ( 'NONE', ( #16473, #17228 ) ) ;
#19662=ORIENTED_EDGE ( 'NONE', *, *, #12855, .F. ) ;
#19666=DIRECTION ( 'NONE',  ( 0.000000000000000000, -1.000000000000000000, -5.286776307738891306E-15 ) ) ;
#19676=PLANE ( 'NONE',  #21620 ) ;
#19678=EDGE_CURVE ( 'NONE', #3554, #21032, #4179, .T. ) ;
#19681=CYLINDRICAL_SURFACE ( 'NONE', #10937, 2.649999999999971934 ) ;
#19688=LINE ( 'NONE', #14403, #8362 ) ;
#19706=ORIENTED_EDGE ( 'NONE', *, *, #16007, .F. ) ;
#19719=EDGE_CURVE ( 'NONE', #14837, #2779, #3396, .T. ) ;
#19744=CARTESIAN_POINT ( 'NONE',  ( -282.6339272673398000, 272.3699028110927429, 145.4976310729378213 ) ) ;
#19745=LINE ( 'NONE', #5140, #11527 ) ;
#19746=CARTESIAN_POINT ( 'NONE',  ( -285.0335297745772323, 269.1488036478618824, -146.2439791848363768 ) ) ;
#19755=DIRECTION ( 'NONE',  ( 0.000000000000000000, -0.000000000000000000, 1.000000000000000000 ) ) ;
#19758=DIRECTION ( 'NONE',  ( -3.495664435217746987E-15, 1.000000000000000000, 0.000000000000000000 ) ) ;
#19762=CARTESIAN_POINT ( 'NONE',  ( -285.2000000000000455, 268.1431883596741841, 146.4301685938042112 ) ) ;
#19763=VECTOR ( 'NONE', #4445, 1000.000000000000000 ) ;
#19774=CARTESIAN_POINT ( 'NONE',  ( 280.8708543776410806, 269.1333820183295416, 146.7350371479513171 ) ) ;
#19776=DIRECTION ( 'NONE',  ( -0.000000000000000000, 1.000000000000000000, -0.000000000000000000 ) ) ;
#19779=EDGE_CURVE ( 'NONE', #14699, #22322, #2749, .T. ) ;
#19786=ORIENTED_EDGE ( 'NONE', *, *, #995, .T. ) ;
#19805=ADVANCED_FACE ( 'NONE', ( #11221 ), #18292, .F. ) ;
#19815=CARTESIAN_POINT ( 'NONE',  ( -280.8089314698395356, 269.2533442688712739, 146.6578961534456482 ) ) ;
#19820=VERTEX_POINT ( 'NONE', #16627 ) ;
#19852=CIRCLE ( 'NONE', #15254, 5.249999999999949374 ) ;
#19854=DIRECTION ( 'NONE',  ( -1.000000000000000000, 0.000000000000000000, -0.000000000000000000 ) ) ;
#19855=DIRECTION ( 'NONE',  ( -0.000000000000000000, -0.000000000000000000, 1.000000000000000000 ) ) ;
#19857=ORIENTED_EDGE ( 'NONE', *, *, #17099, .F. ) ;
#19864=CARTESIAN_POINT ( 'NONE',  ( -280.6847249064869629, 273.0299999999999159, 145.1244295015775947 ) ) ;
#19866=ADVANCED_FACE ( 'NONE', ( #13388 ), #2470, .F. ) ;
#19876=CARTESIAN_POINT ( 'NONE',  ( -281.4928932188134922, -132.2000000000000455, -7.703011046602857601E-15 ) ) ;
#19880=DIRECTION ( 'NONE',  ( -0.000000000000000000, 0.000000000000000000, 1.000000000000000000 ) ) ;
#19882=CIRCLE ( 'NONE', #2134, 2.649999999999971934 ) ;
#19894=LINE ( 'NONE', #21608, #2576 ) ;
#19922=AXIS2_PLACEMENT_3D ( 'NONE', #14323, #46, #18367 ) ;
#19932=FACE_OUTER_BOUND ( 'NONE', #6320, .T. ) ;
#19934=EDGE_CURVE ( 'NONE', #9824, #12957, #11814, .T. ) ;
#19935=FACE_OUTER_BOUND ( 'NONE', #5509, .T. ) ;
#19940=EDGE_LOOP ( 'NONE', ( #8972, #4439, #1360, #15937 ) ) ;
#19941=EDGE_LOOP ( 'NONE', ( #5638, #2236, #23760, #264 ) ) ;
#19944=FACE_OUTER_BOUND ( 'NONE', #7893, .T. ) ;
#19946=LINE ( 'NONE', #18253, #1006 ) ;
#19955=ORIENTED_EDGE ( 'NONE', *, *, #515, .T. ) ;
#19971=AXIS2_PLACEMENT_3D ( 'NONE', #11241, #11347, #18553 ) ;
#19977=CARTESIAN_POINT ( 'NONE',  ( -284.1582675804706355, 270.9956429438695409, 145.8708543776411659 ) ) ;
#19980=EDGE_LOOP ( 'NONE', ( #17836, #1429 ) ) ;
#19984=DIRECTION ( 'NONE',  ( 0.000000000000000000, 0.000000000000000000, -1.000000000000000000 ) ) ;
#19990=AXIS2_PLACEMENT_3D ( 'NONE', #11786, #19215, #9833 ) ;
#19994=CARTESIAN_POINT ( 'NONE',  ( -282.2000000000008981, 30.00000000000101963, -107.6499999999999773 ) ) ;
#20002=ORIENTED_EDGE ( 'NONE', *, *, #21945, .T. ) ;
#20019=CARTESIAN_POINT ( 'NONE',  ( -280.0000000000000568, 269.9999999999999432, -144.9999999999999716 ) ) ;
#20021=CIRCLE ( 'NONE', #12748, 2.649999999999971934 ) ;
#20024=ORIENTED_EDGE ( 'NONE', *, *, #6927, .T. ) ;
#20049=VECTOR ( 'NONE', #1973, 1000.000000000000000 ) ;
#20068=ORIENTED_EDGE ( 'NONE', *, *, #18003, .F. ) ;
#20098=CYLINDRICAL_SURFACE ( 'NONE', #22374, 2.199999999999979750 ) ;
#20102=CARTESIAN_POINT ( 'NONE',  ( -281.7592670532760053, 269.1520027839447948, 145.8708543776411659 ) ) ;
#20120=ORIENTED_EDGE ( 'NONE', *, *, #17902, .F. ) ;
#20151=DIRECTION ( 'NONE',  ( 0.000000000000000000, -1.000000000000000000, -5.286776307738891306E-15 ) ) ;
#20167=PLANE ( 'NONE',  #3043 ) ;
#20169=DIRECTION ( 'NONE',  ( 0.000000000000000000, 0.000000000000000000, -1.000000000000000000 ) ) ;
#20176=FACE_OUTER_BOUND ( 'NONE', #15586, .T. ) ;
#20178=LINE ( 'NONE', #23688, #3741 ) ;
#20185=ORIENTED_EDGE ( 'NONE', *, *, #1350, .F. ) ;
#20186=DIRECTION ( 'NONE',  ( 1.000000000000000000, -3.495664435217746987E-15, -0.000000000000000000 ) ) ;
#20199=ORIENTED_EDGE ( 'NONE', *, *, #787, .F. ) ;
#20205=CARTESIAN_POINT ( 'NONE',  ( 280.0627656775836272, 270.0000000000000000, -145.1452901038202015 ) ) ;
#20210=CARTESIAN_POINT ( 'NONE',  ( 45.00000000000000000, 272.9999999999999432, 0.000000000000000000 ) ) ;
#20211=CARTESIAN_POINT ( 'NONE',  ( -100.0000000000001137, -132.1999999999992212, 147.2000000000013813 ) ) ;
#20215=AXIS2_PLACEMENT_3D ( 'NONE', #8476, #10548, #21498 ) ;
#20238=DIRECTION ( 'NONE',  ( 1.000000000000000000, 0.000000000000000000, -0.000000000000000000 ) ) ;
#20244=CIRCLE ( 'NONE', #9866, 5.199999999999982414 ) ;
#20246=LINE ( 'NONE', #7450, #15533 ) ;
#20248=ORIENTED_EDGE ( 'NONE', *, *, #23141, .F. ) ;
#20256=LINE ( 'NONE', #9306, #18452 ) ;
#20263=CIRCLE ( 'NONE', #21429, 5.249999999999973355 ) ;
#20266=DIRECTION ( 'NONE',  ( 0.000000000000000000, 0.000000000000000000, -1.000000000000000000 ) ) ;
#20268=VERTEX_POINT ( 'NONE', #7515 ) ;
#20278=CARTESIAN_POINT ( 'NONE',  ( 280.3431883596740590, 272.9999999999998295, 145.0627246250092242 ) ) ;
#20284=FACE_OUTER_BOUND ( 'NONE', #3371, .T. ) ;
#20291=LINE ( 'NONE', #2055, #15363 ) ;
#20293=DIRECTION ( 'NONE',  ( 1.000000000000000000, -6.640089860198304064E-16, -0.000000000000000000 ) ) ;
#20303=CARTESIAN_POINT ( 'NONE',  ( -280.0000000000000568, 272.9999999999999432, 145.0000000000000284 ) ) ;
#20307=DIRECTION ( 'NONE',  ( 1.000000000000000000, -0.000000000000000000, -0.000000000000000000 ) ) ;
#20309=EDGE_LOOP ( 'NONE', ( #4792, #2453, #21025, #21446 ) ) ;
#20314=EDGE_CURVE ( 'NONE', #12183, #733, #12323, .T. ) ;
#20315=VECTOR ( 'NONE', #11626, 1000.000000000000000 ) ;
#20316=APPLICATION_CONTEXT ( 'automotive_design' ) ;
#20325=CARTESIAN_POINT ( 'NONE',  ( 280.9955614683501608, 270.4045710003932754, -149.5135885331258692 ) ) ;
#20333=AXIS2_PLACEMENT_3D ( 'NONE', #1619, #17934, #12656 ) ;
#20335=FACE_OUTER_BOUND ( 'NONE', #6140, .T. ) ;
#20340=CIRCLE ( 'NONE', #11529, 5.249999999999991118 ) ;
#20341=CARTESIAN_POINT ( 'NONE',  ( 282.1999999999999318, 269.9999999999999432, 146.4928932188134638 ) ) ;
#20346=CYLINDRICAL_SURFACE ( 'NONE', #6166, 5.249999999999942268 ) ;
#20351=ADVANCED_FACE ( 'NONE', ( #1227 ), #11905, .F. ) ;
#20352=CARTESIAN_POINT ( 'NONE',  ( 280.5743436287469308, 269.9433523009093392, -145.2481149223241061 ) ) ;
#20354=ORIENTED_EDGE ( 'NONE', *, *, #15638, .T. ) ;
#20355=AXIS2_PLACEMENT_3D ( 'NONE', #2689, #21036, #8599 ) ;
#20367=EDGE_LOOP ( 'NONE', ( #22860, #7141 ) ) ;
#20376=ORIENTED_EDGE ( 'NONE', *, *, #5335, .F. ) ;
#20397=ADVANCED_FACE ( 'NONE', ( #15866 ), #9951, .T. ) ;
#20405=CARTESIAN_POINT ( 'NONE',  ( 279.9999999999999432, 272.9999999999999432, 145.0000000000000284 ) ) ;
#20421=AXIS2_PLACEMENT_3D ( 'NONE', #5959, #15985, #4865 ) ;
#20426=EDGE_LOOP ( 'NONE', ( #13568, #3862, #276, #5794 ) ) ;
#20427=CARTESIAN_POINT ( 'NONE',  ( 285.1999999999999886, 268.1431883596741841, -146.4301685938041828 ) ) ;
#20428=ORIENTED_EDGE ( 'NONE', *, *, #6767, .F. ) ;
#20437=ORIENTED_EDGE ( 'NONE', *, *, #1075, .T. ) ;
#20445=CARTESIAN_POINT ( 'NONE',  ( -281.6574776399289703, 269.2538215477172230, 145.8086578304521197 ) ) ;
#20447=ORIENTED_EDGE ( 'NONE', *, *, #19391, .T. ) ;
#20451=CARTESIAN_POINT ( 'NONE',  ( 279.9999999999999432, 273.0299999999999159, 145.0000000000000284 ) ) ;
#20457=CARTESIAN_POINT ( 'NONE',  ( -281.3518577254347406, 272.8327955282141488, -145.2494876630256613 ) ) ;
#20463=DIRECTION ( 'NONE',  ( 1.000000000000000000, -0.000000000000000000, -0.000000000000000000 ) ) ;
#20481=DIRECTION ( 'NONE',  ( -0.000000000000000000, 0.000000000000000000, -1.000000000000000000 ) ) ;
#20483=CARTESIAN_POINT ( 'NONE',  ( 282.0873946496628264, 268.5095819834011195, -146.1815513148989112 ) ) ;
#20492=ADVANCED_FACE ( 'NONE', ( #6904 ), #1806, .T. ) ;
#20509=EDGE_LOOP ( 'NONE', ( #23409, #4576, #2671, #10940 ) ) ;
#20512=EDGE_LOOP ( 'NONE', ( #23676, #16114, #2759, #3274 ) ) ;
#20513=LINE ( 'NONE', #15118, #8676 ) ;
#20520=EDGE_CURVE ( 'NONE', #12822, #13119, #23436, .T. ) ;
#20521=CARTESIAN_POINT ( 'NONE',  ( 287.4000000000013415, -127.0000000000000568, -146.4928932188134070 ) ) ;
#20527=CARTESIAN_POINT ( 'NONE',  ( -282.2000000000010118, 9.787860418609727755E-13, 0.000000000000000000 ) ) ;
#20536=ORIENTED_EDGE ( 'NONE', *, *, #14512, .F. ) ;
#20541=CARTESIAN_POINT ( 'NONE',  ( -281.4928932188134354, 267.8000000000000114, -150.1999999999999318 ) ) ;
#20553=CARTESIAN_POINT ( 'NONE',  ( -280.6220388411722411, 269.5592670532760167, -146.3520027839447835 ) ) ;
#20555=VECTOR ( 'NONE', #4218, 1000.000000000000000 ) ;
#20559=ADVANCED_FACE ( 'NONE', ( #19932 ), #3383, .F. ) ;
#20562=EDGE_CURVE ( 'NONE', #21142, #3965, #19315, .T. ) ;
#20564=CARTESIAN_POINT ( 'NONE',  ( 284.5436892194421148, 270.4188186979286002, 145.9952621458756710 ) ) ;
#20565=CARTESIAN_POINT ( 'NONE',  ( -285.0938770989753834, 269.1689414351989740, -146.2440776823445390 ) ) ;
#20571=VERTEX_POINT ( 'NONE', #22210 ) ;
#20579=DIRECTION ( 'NONE',  ( -3.495664435217746592E-15, -1.000000000000000000, 0.000000000000000000 ) ) ;
#20589=ORIENTED_EDGE ( 'NONE', *, *, #6365, .F. ) ;
#20612=VERTEX_POINT ( 'NONE', #249 ) ;
#20619=EDGE_CURVE ( 'NONE', #13591, #14699, #8094, .T. ) ;
#20621=ORIENTED_EDGE ( 'NONE', *, *, #734, .F. ) ;
#20625=ORIENTED_EDGE ( 'NONE', *, *, #10516, .T. ) ;
#20634=ORIENTED_EDGE ( 'NONE', *, *, #6574, .T. ) ;
#20636=CARTESIAN_POINT ( 'NONE',  ( -280.6222583006965010, 271.9268706878667103, -148.1682701916305973 ) ) ;
#20637=VECTOR ( 'NONE', #14815, 1000.000000000000000 ) ;
#20642=AXIS2_PLACEMENT_3D ( 'NONE', #967, #15724, #6655 ) ;
#20645=FACE_BOUND ( 'NONE', #18374, .T. ) ;
#20646=CARTESIAN_POINT ( 'NONE',  ( -288.2000000000008981, 35.00000000000100897, 105.0000000000000000 ) ) ;
#20654=ADVANCED_FACE ( 'NONE', ( #14999 ), #22342, .T. ) ;
#20658=EDGE_CURVE ( 'NONE', #22534, #20268, #19580, .T. ) ;
#20661=ORIENTED_EDGE ( 'NONE', *, *, #2615, .F. ) ;
#20666=PLANE ( 'NONE',  #14146 ) ;
#20674=CARTESIAN_POINT ( 'NONE',  ( -280.9952621458755857, 268.8927021017107108, -146.8958543268122128 ) ) ;
#20678=AXIS2_PLACEMENT_3D ( 'NONE', #4019, #22498, #5967 ) ;
#20681=CARTESIAN_POINT ( 'NONE',  ( 282.1427398886702917, 268.3758453455903918, 146.2440776823445958 ) ) ;
#20684=VECTOR ( 'NONE', #1213, 1000.000000000000000 ) ;
#20686=VECTOR ( 'NONE', #3143, 1000.000000000000000 ) ;
#20690=EDGE_LOOP ( 'NONE', ( #19786, #8083, #6391, #12975 ) ) ;
#20702=CYLINDRICAL_SURFACE ( 'NONE', #4143, 5.249999999999973355 ) ;
#20722=AXIS2_PLACEMENT_3D ( 'NONE', #23362, #17461, #905 ) ;
#20726=CYLINDRICAL_SURFACE ( 'NONE', #3409, 2.649999999999971934 ) ;
#20734=FACE_BOUND ( 'NONE', #12557, .T. ) ;
#20748=ORIENTED_EDGE ( 'NONE', *, *, #13754, .T. ) ;
#20752=DIRECTION ( 'NONE',  ( 3.495664435217746987E-15, -1.000000000000000000, -0.000000000000000000 ) ) ;
#20761=CARTESIAN_POINT ( 'NONE',  ( 281.4928932188133786, 267.8000000000000114, -147.1999999999999318 ) ) ;
#20764=CARTESIAN_POINT ( 'NONE',  ( 284.9329465209281693, 269.4795879751484904, 146.1810844504668125 ) ) ;
#20765=DIRECTION ( 'NONE',  ( 0.000000000000000000, 0.000000000000000000, -1.000000000000000000 ) ) ;
#20767=VECTOR ( 'NONE', #14414, 1000.000000000000000 ) ;
#20770=DIRECTION ( 'NONE',  ( -3.495664435217746987E-15, -1.000000000000000000, 0.000000000000000000 ) ) ;
#20772=EDGE_CURVE ( 'NONE', #17208, #640, #6619, .T. ) ;
#20776=CARTESIAN_POINT ( 'NONE',  ( 280.6220388411722411, 269.5592670532759598, -146.3520027839447550 ) ) ;
#20784=VECTOR ( 'NONE', #1343, 1000.000000000000000 ) ;
#20787=CARTESIAN_POINT ( 'NONE',  ( 283.0299054689546665, 272.0295083325147516, -145.5908103165959631 ) ) ;
#20791=DIRECTION ( 'NONE',  ( -0.000000000000000000, -0.000000000000000000, 1.000000000000000000 ) ) ;
#20793=ORIENTED_EDGE ( 'NONE', *, *, #5584, .T. ) ;
#20804=CARTESIAN_POINT ( 'NONE',  ( -280.0000000000000000, 269.9697000000000457, -144.9999999999999716 ) ) ;
#20806=EDGE_CURVE ( 'NONE', #22426, #22539, #11169, .T. ) ;
#20818=FACE_OUTER_BOUND ( 'NONE', #5041, .T. ) ;
#20826=AXIS2_PLACEMENT_3D ( 'NONE', #14779, #22475, #5941 ) ;
#20831=CARTESIAN_POINT ( 'NONE',  ( 40.00000000000000000, 100.0000000000000000, -150.2000000000005571 ) ) ;
#20834=CARTESIAN_POINT ( 'NONE',  ( -285.2000000000008981, 35.00000000000100897, 102.3500000000000227 ) ) ;
#20835=ORIENTED_EDGE ( 'NONE', *, *, #11106, .F. ) ;
#20853=AXIS2_PLACEMENT_3D ( 'NONE', #8818, #23549, #13418 ) ;
#20856=CARTESIAN_POINT ( 'NONE',  ( -282.2000000000010687, -19.99999999999898392, 102.3500000000000227 ) ) ;
#20858=EDGE_CURVE ( 'NONE', #19820, #19084, #22155, .T. ) ;
#20860=DIRECTION ( 'NONE',  ( 0.000000000000000000, -3.495664435217746987E-15, 1.000000000000000000 ) ) ;
#20866=CARTESIAN_POINT ( 'NONE',  ( 280.6845057130643113, 271.7107452280322377, 148.4314821058792404 ) ) ;
#20867=DIRECTION ( 'NONE',  ( -1.000000000000000000, -0.000000000000000000, -0.000000000000000000 ) ) ;
#20869=EDGE_LOOP ( 'NONE', ( #12070, #10288, #12923, #22956 ) ) ;
#20870=CARTESIAN_POINT ( 'NONE',  ( 282.1999999999999318, 267.7999999999999545, -146.4928932188133786 ) ) ;
#20885=EDGE_CURVE ( 'NONE', #7573, #5160, #12719, .T. ) ;
#20888=CYLINDRICAL_SURFACE ( 'NONE', #13775, 2.649999999999971934 ) ;
#20895=DIRECTION ( 'NONE',  ( 0.000000000000000000, -1.000000000000000000, 0.000000000000000000 ) ) ;
#20896=PLANE ( 'NONE',  #1519 ) ;
#20912=CARTESIAN_POINT ( 'NONE',  ( -281.4928932188135491, 267.7999999999999545, 150.1999999999999886 ) ) ;
#20920=ORIENTED_EDGE ( 'NONE', *, *, #14807, .F. ) ;
#20921=CARTESIAN_POINT ( 'NONE',  ( -280.6220388411722411, 269.5350371479513569, -146.3333820183295302 ) ) ;
#20927=EDGE_CURVE ( 'NONE', #2779, #21906, #18410, .T. ) ;
#20928=CARTESIAN_POINT ( 'NONE',  ( 280.2880230824754335, 269.9999999999999432, 145.1244266708879707 ) ) ;
#20938=EDGE_CURVE ( 'NONE', #5337, #22099, #1643, .T. ) ;
#20948=VERTEX_POINT ( 'NONE', #7322 ) ;
#20956=DIRECTION ( 'NONE',  ( -0.000000000000000000, -0.000000000000000000, 1.000000000000000000 ) ) ;
#20957=CARTESIAN_POINT ( 'NONE',  ( -40.00000000000000000, 100.0000000000000000, 147.2000000000005855 ) ) ;
#20958=AXIS2_PLACEMENT_3D ( 'NONE', #20957, #15900, #23121 ) ;
#20963=VERTEX_POINT ( 'NONE', #19994 ) ;
#20966=DIRECTION ( 'NONE',  ( -1.000000000000000000, -0.000000000000000000, -0.000000000000000000 ) ) ;
#20972=DIRECTION ( 'NONE',  ( 0.000000000000000000, -3.491481338843133355E-15, 1.000000000000000000 ) ) ;
#20975=EDGE_CURVE ( 'NONE', #5337, #17412, #16168, .T. ) ;
#20976=ORIENTED_EDGE ( 'NONE', *, *, #3968, .F. ) ;
#20982=CARTESIAN_POINT ( 'NONE',  ( 281.4928932188134354, 267.8000000000000114, -147.1999999999999318 ) ) ;
#20989=DIRECTION ( 'NONE',  ( 0.000000000000000000, -1.000000000000000000, 0.000000000000000000 ) ) ;
#20990=LINE ( 'NONE', #22668, #19763 ) ;
#20995=DIRECTION ( 'NONE',  ( -0.000000000000000000, 1.000000000000000000, -0.000000000000000000 ) ) ;
#20996=CARTESIAN_POINT ( 'NONE',  ( -287.4000000000014552, -127.0000000000000568, -146.4928932188134070 ) ) ;
#20997=AXIS2_PLACEMENT_3D ( 'NONE', #22554, #2517, #14985 ) ;
#21000=CARTESIAN_POINT ( 'NONE',  ( 0.000000000000000000, 0.000000000000000000, -150.2000000000008981 ) ) ;
#21003=CARTESIAN_POINT ( 'NONE',  ( 312.2000000000013529, -129.2000000000000455, -146.4928932188134070 ) ) ;
#21025=ORIENTED_EDGE ( 'NONE', *, *, #12899, .F. ) ;
#21030=CARTESIAN_POINT ( 'NONE',  ( -280.8708543776413080, 270.9956429438695409, 149.1582675804705218 ) ) ;
#21032=VERTEX_POINT ( 'NONE', #9865 ) ;
#21035=FACE_OUTER_BOUND ( 'NONE', #20309, .T. ) ;
#21036=DIRECTION ( 'NONE',  ( 0.000000000000000000, 0.000000000000000000, -1.000000000000000000 ) ) ;
#21037=VECTOR ( 'NONE', #11693, 1000.000000000000000 ) ;
#21044=ORIENTED_EDGE ( 'NONE', *, *, #20772, .T. ) ;
#21062=VERTEX_POINT ( 'NONE', #17221 ) ;
#21096=AXIS2_PLACEMENT_3D ( 'NONE', #4955, #15718, #12493 ) ;
#21102=PLANE ( 'NONE',  #13497 ) ;
#21107=CARTESIAN_POINT ( 'NONE',  ( -280.2481149223241346, 269.9433523009093392, -145.5743436287470161 ) ) ;
#21114=FACE_OUTER_BOUND ( 'NONE', #13192, .T. ) ;
#21132=CYLINDRICAL_SURFACE ( 'NONE', #23505, 5.249999999999942268 ) ;
#21134=VECTOR ( 'NONE', #21457, 1000.000000000000000 ) ;
#21142=VERTEX_POINT ( 'NONE', #21424 ) ;
#21143=CARTESIAN_POINT ( 'NONE',  ( 45.00000000000000000, 269.9999999999999432, 0.000000000000000000 ) ) ;
#21149=CARTESIAN_POINT ( 'NONE',  ( -280.0000000000000568, 269.9696999999999889, 145.0000000000000284 ) ) ;
#21169=DIRECTION ( 'NONE',  ( 0.000000000000000000, -3.491481338843133355E-15, 1.000000000000000000 ) ) ;
#21173=DIRECTION ( 'NONE',  ( 0.000000000000000000, -1.000000000000000000, 0.000000000000000000 ) ) ;
#21175=CARTESIAN_POINT ( 'NONE',  ( -281.9223300543794721, 268.9079617568158938, -145.9952621458756141 ) ) ;
#21195=ORIENTED_EDGE ( 'NONE', *, *, #8341, .F. ) ;
#21197=VECTOR ( 'NONE', #8263, 1000.000000000000000 ) ;
#21212=CARTESIAN_POINT ( 'NONE',  ( 287.4000000000013415, -129.2000000000000455, 146.4928932188134638 ) ) ;
#21240=CARTESIAN_POINT ( 'NONE',  ( -285.2000000000006708, 90.00000000000100897, 34.99999999999999289 ) ) ;
#21244=CARTESIAN_POINT ( 'NONE',  ( 279.9999999999999432, 273.0299999999999159, 145.0000000000000284 ) ) ;
#21261=LINE ( 'NONE', #14040, #21525 ) ;
#21263=EDGE_CURVE ( 'NONE', #21906, #13397, #17563, .T. ) ;
#21264=ORIENTED_EDGE ( 'NONE', *, *, #21277, .T. ) ;
#21274=EDGE_CURVE ( 'NONE', #19104, #22322, #22737, .T. ) ;
#21275=CARTESIAN_POINT ( 'NONE',  ( -280.2488155364689533, 272.8938770989752811, 146.3689414351990763 ) ) ;
#21277=EDGE_CURVE ( 'NONE', #19820, #4309, #12652, .T. ) ;
#21282=CARTESIAN_POINT ( 'NONE',  ( -280.0000000000000568, 269.9999999999999432, 145.0000000000000284 ) ) ;
#21288=ADVANCED_FACE ( 'NONE', ( #14553 ), #18049, .F. ) ;
#21291=VERTEX_POINT ( 'NONE', #16605 ) ;
#21298=ORIENTED_EDGE ( 'NONE', *, *, #5592, .F. ) ;
#21302=DIRECTION ( 'NONE',  ( -1.000000000000000000, 3.495664435217746987E-15, 0.000000000000000000 ) ) ;
#21306=FACE_OUTER_BOUND ( 'NONE', #10965, .T. ) ;
#21315=DIRECTION ( 'NONE',  ( 1.000000000000000000, 0.000000000000000000, -0.000000000000000000 ) ) ;
#21327=CARTESIAN_POINT ( 'NONE',  ( 45.24999999999994316, 100.0000000000000000, 147.2000000000005855 ) ) ;
#21329=CARTESIAN_POINT ( 'NONE',  ( -285.2000000000000455, 268.1431883566700662, -146.4301685943532618 ) ) ;
#21331=ORIENTED_EDGE ( 'NONE', *, *, #1321, .F. ) ;
#21338=CARTESIAN_POINT ( 'NONE',  ( 45.00000000000000000, 272.9999999999999432, 0.000000000000000000 ) ) ;
#21343=CARTESIAN_POINT ( 'NONE',  ( -285.2000000000000455, 267.7999999999999545, 146.4928932188134354 ) ) ;
#21346=CARTESIAN_POINT ( 'NONE',  ( -280.6839617489741840, 269.4578961534455175, -146.4533442688710920 ) ) ;
#21350=B_SPLINE_SURFACE_WITH_KNOTS ( 'NONE', 1, 3, ( 
 ( #13193, #10764, #5652, #23649, #18109, #1415, #1670, #16415, #9051, #14494 ),
 ( #7458, #22181, #16762, #7578, #14969, #7110, #1564, #8948, #16305, #11473 ),
 ( #17126, #9525, #22897, #22540, #17019, #6259, #472, #13778, #15326, #20870 ),
 ( #4323, #19156, #22427, #5888, #11612, #7825, #2619, #15209, #13665, #22795 ) ),
 .UNSPECIFIED., .F., .F., .F.,
 ( 2, 1, 1, 2 ),
 ( 4, 2, 2, 2, 4 ),
 ( -0.01000000000000000021, 0.000000000000000000, 1.000000000000000000, 1.010099999999999998 ),
 ( 0.000000000000000000, 0.2500000000000000000, 0.5000000000000000000, 0.7500000000000000000, 1.000000000000000000 ),
 .UNSPECIFIED. ) ;
#21354=LINE ( 'NONE', #2983, #23293 ) ;
#21356=ORIENTED_EDGE ( 'NONE', *, *, #4889, .F. ) ;
#21360=FACE_OUTER_BOUND ( 'NONE', #22923, .T. ) ;
#21361=ORIENTED_EDGE ( 'NONE', *, *, #10326, .T. ) ;
#21365=CARTESIAN_POINT ( 'NONE',  ( -281.1807969192698238, 269.4810649015077502, -149.9324007871373112 ) ) ;
#21373=ADVANCED_FACE ( 'NONE', ( #7163 ), #10840, .F. ) ;
#21377=VECTOR ( 'NONE', #15651, 1000.000000000000000 ) ;
#21378=DIRECTION ( 'NONE',  ( -0.000000000000000000, -0.000000000000000000, 1.000000000000000000 ) ) ;
#21388=DIRECTION ( 'NONE',  ( 0.000000000000000000, -3.491481338843133355E-15, -1.000000000000000000 ) ) ;
#21390=CARTESIAN_POINT ( 'NONE',  ( 40.00000000000000000, 100.0000000000000000, 147.2000000000005855 ) ) ;
#21398=DIRECTION ( 'NONE',  ( -0.000000000000000000, 1.000000000000000000, 0.000000000000000000 ) ) ;
#21400=ADVANCED_FACE ( 'NONE', ( #5480 ), #1093, .F. ) ;
#21401=CARTESIAN_POINT ( 'NONE',  ( -280.0000000000000568, 272.9999999999999432, -144.9999999999999716 ) ) ;
#21402=EDGE_CURVE ( 'NONE', #8982, #5006, #17561, .T. ) ;
#21417=VERTEX_POINT ( 'NONE', #17895 ) ;
#21420=CARTESIAN_POINT ( 'NONE',  ( -281.1810844504668125, 269.4795879751483767, 149.9329465209280272 ) ) ;
#21424=CARTESIAN_POINT ( 'NONE',  ( -282.2000000000000455, 267.7999999999999545, -146.4928932188134354 ) ) ;
#21426=DIRECTION ( 'NONE',  ( -1.000000000000000000, 3.495664435217746987E-15, 0.000000000000000000 ) ) ;
#21429=AXIS2_PLACEMENT_3D ( 'NONE', #21143, #2888, #23426 ) ;
#21446=ORIENTED_EDGE ( 'NONE', *, *, #7831, .F. ) ;
#21454=DIRECTION ( 'NONE',  ( -0.000000000000000000, 0.000000000000000000, -1.000000000000000000 ) ) ;
#21457=DIRECTION ( 'NONE',  ( -1.000000000000000000, 0.000000000000000000, 0.000000000000000000 ) ) ;
#21466=VERTEX_POINT ( 'NONE', #10306 ) ;
#21471=CARTESIAN_POINT ( 'NONE',  ( 280.6220388411721274, 271.9822575857424454, 148.2140793454688037 ) ) ;
#21480=DIRECTION ( 'NONE',  ( 0.000000000000000000, -3.495664435217746987E-15, 1.000000000000000000 ) ) ;
#21486=CARTESIAN_POINT ( 'NONE',  ( -280.9953931959807392, 270.4054396500289954, -149.5132312761074047 ) ) ;
#21488=DIRECTION ( 'NONE',  ( -1.000000000000000000, -0.000000000000000000, -0.000000000000000000 ) ) ;
#21489=ORIENTED_EDGE ( 'NONE', *, *, #7973, .F. ) ;
#21493=VECTOR ( 'NONE', #23149, 1000.000000000000000 ) ;
#21496=CARTESIAN_POINT ( 'NONE',  ( -280.0000000000000568, 272.9999999999999432, -144.9999999999999716 ) ) ;
#21498=DIRECTION ( 'NONE',  ( 0.000000000000000000, 0.000000000000000000, 1.000000000000000000 ) ) ;
#21500=EDGE_CURVE ( 'NONE', #17208, #15945, #8494, .T. ) ;
#21525=VECTOR ( 'NONE', #4710, 1000.000000000000000 ) ;
#21538=DIRECTION ( 'NONE',  ( -0.000000000000000000, 1.000000000000000000, 0.000000000000000000 ) ) ;
#21540=DIRECTION ( 'NONE',  ( 3.700743415417189520E-15, 1.000000000000000000, 0.000000000000000000 ) ) ;
#21573=ORIENTED_EDGE ( 'NONE', *, *, #9786, .F. ) ;
#21579=CARTESIAN_POINT ( 'NONE',  ( 0.000000000000000000, 269.9999999999999432, 0.000000000000000000 ) ) ;
#21580=EDGE_CURVE ( 'NONE', #9425, #20571, #12265, .T. ) ;
#21586=DIRECTION ( 'NONE',  ( 0.000000000000000000, 0.000000000000000000, 1.000000000000000000 ) ) ;
#21589=DIRECTION ( 'NONE',  ( -1.000000000000000000, 3.495664435217746987E-15, 0.000000000000000000 ) ) ;
#21598=CARTESIAN_POINT ( 'NONE',  ( 279.9999999999999432, 269.9999999999999432, 145.0000000000000284 ) ) ;
#21602=AXIS2_PLACEMENT_3D ( 'NONE', #18235, #11274, #9324 ) ;
#21606=ORIENTED_EDGE ( 'NONE', *, *, #16312, .T. ) ;
#21607=CARTESIAN_POINT ( 'NONE',  ( 280.4976310729377360, 269.6958543268121957, 146.0927021017107563 ) ) ;
#21608=CARTESIAN_POINT ( 'NONE',  ( -45.00000000000000000, 272.9999999999999432, -5.249999999999973355 ) ) ;
#21615=CARTESIAN_POINT ( 'NONE',  ( -40.00000000000000000, 100.0000000000000000, 150.2000000000009550 ) ) ;
#21620=AXIS2_PLACEMENT_3D ( 'NONE', #6516, #12365, #3136 ) ;
#21624=CARTESIAN_POINT ( 'NONE',  ( -282.2000000000007276, 75.00000000000098055, 90.00000000000000000 ) ) ;
#21628=CARTESIAN_POINT ( 'NONE',  ( -285.2000000000006708, 90.00000000000100897, 34.99999999999999289 ) ) ;
#21630=ORIENTED_EDGE ( 'NONE', *, *, #23317, .T. ) ;
#21633=ORIENTED_EDGE ( 'NONE', *, *, #2547, .T. ) ;
#21645=FACE_OUTER_BOUND ( 'NONE', #1453, .T. ) ;
#21649=EDGE_LOOP ( 'NONE', ( #12688, #13262, #12905, #4346 ) ) ;
#21652=CARTESIAN_POINT ( 'NONE',  ( 99.99999999999987210, -132.1999999999993634, 147.2000000000013813 ) ) ;
#21655=ORIENTED_EDGE ( 'NONE', *, *, #19525, .T. ) ;
#21660=ORIENTED_EDGE ( 'NONE', *, *, #5467, .F. ) ;
#21665=CARTESIAN_POINT ( 'NONE',  ( -280.9020829022175576, 270.8299054689547347, 149.2295083325148539 ) ) ;
#21678=ORIENTED_EDGE ( 'NONE', *, *, #17010, .F. ) ;
#21684=CARTESIAN_POINT ( 'NONE',  ( -280.2840560642351875, 269.9696999999999889, 145.1244266425809712 ) ) ;
#21686=CARTESIAN_POINT ( 'NONE',  ( -284.9329465209281125, 269.4795879751482630, -146.1810844504667557 ) ) ;
#21690=FACE_OUTER_BOUND ( 'NONE', #12168, .T. ) ;
#21691=DIRECTION ( 'NONE',  ( 0.000000000000000000, 1.000000000000000000, 4.183096374613631247E-18 ) ) ;
#21706=ORIENTED_EDGE ( 'NONE', *, *, #16669, .T. ) ;
#21709=ADVANCED_FACE ( 'NONE', ( #21645 ), #5101, .F. ) ;
#21718=ADVANCED_FACE ( 'NONE', ( #14416 ), #3388, .F. ) ;
#21732=AXIS2_PLACEMENT_3D ( 'NONE', #4878, #23, #8517 ) ;
#21737=DIRECTION ( 'NONE',  ( 0.000000000000000000, 0.000000000000000000, -1.000000000000000000 ) ) ;
#21741=AXIS2_PLACEMENT_3D ( 'NONE', #6393, #15836, #4581 ) ;
#21747=ADVANCED_FACE ( 'NONE', ( #20645, #502, #11511, #139, #18707, #3873, #7752, #4100, #14881, #22214 ), #9805, .F. ) ;
#21753=ORIENTED_EDGE ( 'NONE', *, *, #10824, .T. ) ;
#21778=LINE ( 'NONE', #3533, #13094 ) ;
#21781=DIRECTION ( 'NONE',  ( -1.000000000000000000, 3.495664435217746592E-15, -0.000000000000000000 ) ) ;
#21790=EDGE_CURVE ( 'NONE', #10284, #15178, #11283, .T. ) ;
#21791=CARTESIAN_POINT ( 'NONE',  ( -284.5699028110928452, 270.4339272673396977, 145.9952621458756425 ) ) ;
#21815=LINE ( 'NONE', #14829, #17260 ) ;
#21816=CARTESIAN_POINT ( 'NONE',  ( -281.4928932188135491, -132.2000000000000455, 7.703011046602857601E-15 ) ) ;
#21822=CARTESIAN_POINT ( 'NONE',  ( 281.2440776823444253, 269.1689414351989740, 150.0938770989752982 ) ) ;
#21829=ORIENTED_EDGE ( 'NONE', *, *, #17842, .F. ) ;
#21831=DIRECTION ( 'NONE',  ( -0.000000000000000000, -0.000000000000000000, 1.000000000000000000 ) ) ;
#21838=ORIENTED_EDGE ( 'NONE', *, *, #20658, .T. ) ;
#21839=AXIS2_PLACEMENT_3D ( 'NONE', #23498, #9007, #16371 ) ;
#21846=CARTESIAN_POINT ( 'NONE',  ( -282.2000000000007276, 75.00000000000098055, 90.00000000000000000 ) ) ;
#21849=CARTESIAN_POINT ( 'NONE',  ( 312.2000000000013529, -132.2000000000000455, -146.4928932188134070 ) ) ;
#21869=LINE ( 'NONE', #21652, #23438 ) ;
#21870=EDGE_CURVE ( 'NONE', #11281, #20963, #2970, .T. ) ;
#21880=VERTEX_POINT ( 'NONE', #5294 ) ;
#21882=VERTEX_POINT ( 'NONE', #16650 ) ;
#21885=( LENGTH_UNIT ( ) NAMED_UNIT ( * ) SI_UNIT ( .MILLI., .METRE. ) );
#21887=DIRECTION ( 'NONE',  ( -1.000000000000000000, 3.495664435217746987E-15, 0.000000000000000000 ) ) ;
#21896=DIRECTION ( 'NONE',  ( 0.000000000000000000, 0.000000000000000000, -1.000000000000000000 ) ) ;
#21903=CARTESIAN_POINT ( 'NONE',  ( -281.1079617568159961, 269.7223300543793698, 145.4976310729378213 ) ) ;
#21905=CARTESIAN_POINT ( 'NONE',  ( 280.3120962995436116, 272.7324007871372373, -146.6810649015076535 ) ) ;
#21906=VERTEX_POINT ( 'NONE', #22177 ) ;
#21913=ORIENTED_EDGE ( 'NONE', *, *, #7984, .F. ) ;
#21917=CARTESIAN_POINT ( 'NONE',  ( 0.000000000000000000, -132.2000000000000455, 177.2000000000014097 ) ) ;
#21918=CARTESIAN_POINT ( 'NONE',  ( -288.2000000000011255, -29.99999999999898037, -107.6499999999999631 ) ) ;
#21919=DIRECTION ( 'NONE',  ( 1.000000000000000000, -3.495664435217746987E-15, -0.000000000000000000 ) ) ;
#21921=CIRCLE ( 'NONE', #10396, 35.00000000000000711 ) ;
#21924=EDGE_LOOP ( 'NONE', ( #13856, #17231, #17237, #7889 ) ) ;
#21926=PLANE ( 'NONE',  #4530 ) ;
#21928=EDGE_LOOP ( 'NONE', ( #6824, #20748, #12577, #4946 ) ) ;
#21930=B_SPLINE_SURFACE_WITH_KNOTS ( 'NONE', 1, 3, ( 
 ( #12445, #19864, #7303, #19744, #5490, #1734, #21791, #16264, #3314, #1625 ),
 ( #8774, #16022, #3549, #10721, #18061, #19977, #18280, #7173, #9124, #16479 ),
 ( #15462, #6961, #12800, #21903, #23606, #20102, #14351, #14695, #12902, #7065 ),
 ( #10490, #21684, #17942, #8649, #3436, #6828, #5378, #12664, #14230, #5139 ) ),
 .UNSPECIFIED., .F., .F., .F.,
 ( 2, 1, 1, 2 ),
 ( 4, 2, 2, 2, 4 ),
 ( -0.01000000000000000021, 0.000000000000000000, 1.000000000000000000, 1.010099999999999998 ),
 ( 0.000000000000000000, 0.2500000000000000000, 0.5000000000000000000, 0.7500000000000000000, 1.000000000000000000 ),
 .UNSPECIFIED. ) ;
#21932=LINE ( 'NONE', #10989, #13175 ) ;
#21937=CIRCLE ( 'NONE', #1119, 2.199999999999979750 ) ;
#21939=CARTESIAN_POINT ( 'NONE',  ( -281.4928932188135491, -132.2000000000000455, 152.4000000000014268 ) ) ;
#21942=DIRECTION ( 'NONE',  ( 0.000000000000000000, 1.000000000000000000, 0.000000000000000000 ) ) ;
#21945=EDGE_CURVE ( 'NONE', #15324, #3965, #14386, .T. ) ;
#21946=CARTESIAN_POINT ( 'NONE',  ( 281.4928932188134354, -127.0000000000000568, -147.2000000000013245 ) ) ;
#21952=ORIENTED_EDGE ( 'NONE', *, *, #1972, .T. ) ;
#21970=FACE_OUTER_BOUND ( 'NONE', #23665, .T. ) ;
#21977=ADVANCED_FACE ( 'NONE', ( #1665 ), #7348, .F. ) ;
#21981=ORIENTED_EDGE ( 'NONE', *, *, #22749, .F. ) ;
#21987=LINE ( 'NONE', #20761, #22506 ) ;
#21995=ORIENTED_EDGE ( 'NONE', *, *, #995, .F. ) ;
#21998=DIRECTION ( 'NONE',  ( 1.000000000000000000, -6.640089860198304064E-16, -0.000000000000000000 ) ) ;
#21999=DIRECTION ( 'NONE',  ( -1.000000000000000000, 0.000000000000000000, -0.000000000000000000 ) ) ;
#22001=LINE ( 'NONE', #8979, #6795 ) ;
#22005=EDGE_CURVE ( 'NONE', #16905, #15299, #12565, .T. ) ;
#22015=ADVANCED_FACE ( 'NONE', ( #10502 ), #4794, .T. ) ;
#22022=VERTEX_POINT ( 'NONE', #17590 ) ;
#22030=FACE_OUTER_BOUND ( 'NONE', #18120, .T. ) ;
#22043=FACE_BOUND ( 'NONE', #3998, .T. ) ;
#22051=CARTESIAN_POINT ( 'NONE',  ( 40.00000000000000000, 100.0000000000000000, 150.2000000000009550 ) ) ;
#22063=CARTESIAN_POINT ( 'NONE',  ( -100.0000000000001137, -132.2000000000001592, -113.4834095219707848 ) ) ;
#22076=LINE ( 'NONE', #5546, #16750 ) ;
#22085=EDGE_CURVE ( 'NONE', #16256, #640, #18075, .T. ) ;
#22086=CYLINDRICAL_SURFACE ( 'NONE', #12009, 5.249999999999973355 ) ;
#22088=EDGE_CURVE ( 'NONE', #67, #21882, #2849, .T. ) ;
#22090=CARTESIAN_POINT ( 'NONE',  ( -281.7502846751312404, 269.1405375976306686, -145.8716261326569565 ) ) ;
#22099=VERTEX_POINT ( 'NONE', #7078 ) ;
#22103=CARTESIAN_POINT ( 'NONE',  ( 280.6220388411722411, 269.5350371479513001, -146.3333820183295302 ) ) ;
#22108=ORIENTED_EDGE ( 'NONE', *, *, #12374, .T. ) ;
#22110=ORIENTED_EDGE ( 'NONE', *, *, #18284, .T. ) ;
#22111=CARTESIAN_POINT ( 'NONE',  ( -282.2000000000012960, -74.99999999999899103, -90.00000000000000000 ) ) ;
#22112=CARTESIAN_POINT ( 'NONE',  ( -280.0000000000000000, 270.0000000000000000, -144.9999999999999716 ) ) ;
#22116=VERTEX_POINT ( 'NONE', #5051 ) ;
#22117=CARTESIAN_POINT ( 'NONE',  ( -280.0627246250094800, 273.0000000000000000, 145.3431883596743148 ) ) ;
#22120=EDGE_CURVE ( 'NONE', #5795, #22646, #20340, .T. ) ;
#22139=VECTOR ( 'NONE', #6447, 1000.000000000000000 ) ;
#22141=CARTESIAN_POINT ( 'NONE',  ( 281.2439791848364052, 269.1488036478620529, -150.0335297745770902 ) ) ;
#22145=ORIENTED_EDGE ( 'NONE', *, *, #2812, .T. ) ;
#22151=DIRECTION ( 'NONE',  ( -1.000000000000000000, -0.000000000000000000, -0.000000000000000000 ) ) ;
#22152=CARTESIAN_POINT ( 'NONE',  ( 281.4928932188134354, 267.8000000000000114, -150.1999999999999318 ) ) ;
#22155=LINE ( 'NONE', #9141, #7666 ) ;
#22157=CARTESIAN_POINT ( 'NONE',  ( -288.2000000000008981, 30.00000000000101963, -102.3500000000000369 ) ) ;
#22159=VERTEX_POINT ( 'NONE', #22152 ) ;
#22160=DIRECTION ( 'NONE',  ( 3.495664435217746987E-15, 1.000000000000000000, -0.000000000000000000 ) ) ;
#22165=FACE_OUTER_BOUND ( 'NONE', #6898, .T. ) ;
#22170=CARTESIAN_POINT ( 'NONE',  ( 280.2905802150185082, 269.9999999999999432, -145.1255313583546922 ) ) ;
#22177=CARTESIAN_POINT ( 'NONE',  ( -100.0000000000001137, -129.2000000000000455, 152.4000000000014268 ) ) ;
#22181=CARTESIAN_POINT ( 'NONE',  ( 280.6807971656550080, 272.9999999999999432, -145.1244294735508902 ) ) ;
#22196=DIRECTION ( 'NONE',  ( 0.000000000000000000, 1.000000000000000000, 0.000000000000000000 ) ) ;
#22209=CARTESIAN_POINT ( 'NONE',  ( -281.4928932188134354, -127.0000000000000568, -152.4000000000012847 ) ) ;
#22210=CARTESIAN_POINT ( 'NONE',  ( -282.2000000000014666, -127.0000000000000568, -146.4928932188134070 ) ) ;
#22212=CARTESIAN_POINT ( 'NONE',  ( 285.2000000000013529, -127.0000000000000568, -146.4928932188134070 ) ) ;
#22214=FACE_BOUND ( 'NONE', #8232, .T. ) ;
#22215=LINE ( 'NONE', #3874, #2044 ) ;
#22221=AXIS2_PLACEMENT_3D ( 'NONE', #12130, #6532, #12025 ) ;
#22238=CIRCLE ( 'NONE', #23017, 35.00000000000000711 ) ;
#22239=CARTESIAN_POINT ( 'NONE',  ( -280.7774350431396897, 271.3570580646226063, 148.7968359015656574 ) ) ;
#22243=CARTESIAN_POINT ( 'NONE',  ( -280.2905802150187355, 270.0000000000000000, 145.1255313583548059 ) ) ;
#22249=CARTESIAN_POINT ( 'NONE',  ( 282.1999999999999318, 267.7999999999999545, 146.4928932188134922 ) ) ;
#22255=AXIS2_PLACEMENT_3D ( 'NONE', #8862, #21999, #1238 ) ;
#22264=ORIENTED_EDGE ( 'NONE', *, *, #23033, .T. ) ;
#22266=LINE ( 'NONE', #17981, #14495 ) ;
#22283=DIRECTION ( 'NONE',  ( 1.000000000000000000, 0.000000000000000000, 0.000000000000000000 ) ) ;
#22287=CARTESIAN_POINT ( 'NONE',  ( 282.1999999999999886, 267.9452901038201844, -146.4301275412296945 ) ) ;
#22289=ADVANCED_FACE ( 'NONE', ( #2588 ), #20702, .F. ) ;
#22298=CARTESIAN_POINT ( 'NONE',  ( 7.703011046602857601E-15, -132.2000000000000455, 0.000000000000000000 ) ) ;
#22303=CYLINDRICAL_SURFACE ( 'NONE', #3062, 35.00000000000000711 ) ;
#22310=EDGE_LOOP ( 'NONE', ( #15810, #887, #20354, #23147 ) ) ;
#22311=ORIENTED_EDGE ( 'NONE', *, *, #22088, .T. ) ;
#22322=VERTEX_POINT ( 'NONE', #4032 ) ;
#22323=CARTESIAN_POINT ( 'NONE',  ( -45.24999999999994316, 100.0000000000000000, -147.2000000000005571 ) ) ;
#22333=AXIS2_PLACEMENT_3D ( 'NONE', #14076, #22817, #15488 ) ;
#22338=DIRECTION ( 'NONE',  ( -1.000000000000000000, 0.000000000000000000, -0.000000000000000000 ) ) ;
#22340=DIRECTION ( 'NONE',  ( 0.000000000000000000, 0.000000000000000000, 1.000000000000000000 ) ) ;
#22342=CYLINDRICAL_SURFACE ( 'NONE', #5324, 5.199999999999982414 ) ;
#22344=EDGE_CURVE ( 'NONE', #12593, #2692, #17094, .T. ) ;
#22345=CARTESIAN_POINT ( 'NONE',  ( -45.24999999999994316, 100.0000000000000000, 150.2000000000009550 ) ) ;
#22354=CARTESIAN_POINT ( 'NONE',  ( 281.4928932188134354, 267.8000000000000114, -150.1999999999999318 ) ) ;
#22361=CARTESIAN_POINT ( 'NONE',  ( 285.0327955282141374, 269.1518577254344677, -146.2434055557878025 ) ) ;
#22374=AXIS2_PLACEMENT_3D ( 'NONE', #14689, #16361, #21896 ) ;
#22379=CARTESIAN_POINT ( 'NONE',  ( -280.4976310729378497, 272.3436892194421262, -147.6188186979286741 ) ) ;
#22385=CARTESIAN_POINT ( 'NONE',  ( 285.1999999999999318, 267.7999999999999545, 146.4928932188134922 ) ) ;
#22386=LINE ( 'NONE', #9725, #2549 ) ;
#22391=ORIENTED_EDGE ( 'NONE', *, *, #14682, .F. ) ;
#22394=CARTESIAN_POINT ( 'NONE',  ( 281.4928932188133786, 267.7999999999999545, 150.1999999999999886 ) ) ;
#22395=CARTESIAN_POINT ( 'NONE',  ( 279.9999999999999432, 267.7999999999999545, 150.1999999999999886 ) ) ;
#22408=ORIENTED_EDGE ( 'NONE', *, *, #14082, .F. ) ;
#22411=CYLINDRICAL_SURFACE ( 'NONE', #8497, 5.249999999999942268 ) ;
#22414=ORIENTED_EDGE ( 'NONE', *, *, #14807, .T. ) ;
#22418=VERTEX_POINT ( 'NONE', #14208 ) ;
#22419=CARTESIAN_POINT ( 'NONE',  ( 281.4928932188134354, -132.2000000000000455, -152.4000000000013131 ) ) ;
#22423=CARTESIAN_POINT ( 'NONE',  ( 280.8082263737021549, 271.2379565153279373, 148.9159870726003874 ) ) ;
#22426=VERTEX_POINT ( 'NONE', #8888 ) ;
#22427=CARTESIAN_POINT ( 'NONE',  ( 280.5679143846942907, 269.9132285165672442, -145.2488155364688680 ) ) ;
#22429=DIRECTION ( 'NONE',  ( 0.000000000000000000, -1.000000000000000000, 0.000000000000000000 ) ) ;
#22434=CARTESIAN_POINT ( 'NONE',  ( -100.0000000000001137, -132.1999999999999602, -113.4834095219707848 ) ) ;
#22435=CARTESIAN_POINT ( 'NONE',  ( 282.1999999999999318, 267.7999999999999545, -144.9999999999999716 ) ) ;
#22441=DIRECTION ( 'NONE',  ( -1.000000000000000000, -0.000000000000000000, -0.000000000000000000 ) ) ;
#22448=LINE ( 'NONE', #604, #7501 ) ;
#22455=DIRECTION ( 'NONE',  ( 0.000000000000000000, -1.000000000000000000, 0.000000000000000000 ) ) ;
#22465=CARTESIAN_POINT ( 'NONE',  ( 287.4000000000013415, -129.2000000000000455, -146.4928932188134070 ) ) ;
#22466=CARTESIAN_POINT ( 'NONE',  ( 280.8708543776411943, 270.9956429438695977, -149.1582675804704650 ) ) ;
#22468=DIRECTION ( 'NONE',  ( 0.000000000000000000, -1.000000000000000000, 0.000000000000000000 ) ) ;
#22475=DIRECTION ( 'NONE',  ( -0.000000000000000000, -0.000000000000000000, 1.000000000000000000 ) ) ;
#22478=ORIENTED_EDGE ( 'NONE', *, *, #16790, .T. ) ;
#22488=CARTESIAN_POINT ( 'NONE',  ( -280.8708543776411943, 271.0140793454687582, -149.1822575857424624 ) ) ;
#22493=CARTESIAN_POINT ( 'NONE',  ( -281.4928932188134354, -132.2000000000000455, -177.2000000000013529 ) ) ;
#22494=CARTESIAN_POINT ( 'NONE',  ( 285.1999999999999318, 268.4807971656551331, 146.3684637452625168 ) ) ;
#22497=DIRECTION ( 'NONE',  ( -0.000000000000000000, 1.000000000000000000, 3.495664435217746987E-15 ) ) ;
#22498=DIRECTION ( 'NONE',  ( -1.000000000000000000, 0.000000000000000000, 0.000000000000000000 ) ) ;
#22504=ORIENTED_EDGE ( 'NONE', *, *, #17902, .T. ) ;
#22506=VECTOR ( 'NONE', #9688, 1000.000000000000000 ) ;
#22518=VERTEX_POINT ( 'NONE', #6589 ) ;
#22520=CARTESIAN_POINT ( 'NONE',  ( -285.2000000000008981, 30.00000000000101963, -107.6499999999999773 ) ) ;
#22527=CARTESIAN_POINT ( 'NONE',  ( 40.00000000000000000, 100.0000000000000000, -150.2000000000005571 ) ) ;
#22534=VERTEX_POINT ( 'NONE', #13004 ) ;
#22539=VERTEX_POINT ( 'NONE', #18266 ) ;
#22540=CARTESIAN_POINT ( 'NONE',  ( 281.1079617568158824, 269.7223300543793698, -145.4976310729377644 ) ) ;
#22549=EDGE_LOOP ( 'NONE', ( #751, #17451, #1099, #11020 ) ) ;
#22554=CARTESIAN_POINT ( 'NONE',  ( 287.4000000000013415, -127.0000000000000568, -146.4928932188134070 ) ) ;
#22574=EDGE_CURVE ( 'NONE', #22842, #8989, #21778, .T. ) ;
#22580=EDGE_CURVE ( 'NONE', #11487, #15145, #4186, .T. ) ;
#22584=CARTESIAN_POINT ( 'NONE',  ( 279.9999999999999432, 270.0000000000000000, -144.9999999999999716 ) ) ;
#22590=CARTESIAN_POINT ( 'NONE',  ( 280.6816199723481873, 272.9663417894422537, -145.1245861693739130 ) ) ;
#22591=ORIENTED_EDGE ( 'NONE', *, *, #18455, .T. ) ;
#22605=CARTESIAN_POINT ( 'NONE',  ( -281.3684637452625452, 268.4807971656549626, -150.1999999999999602 ) ) ;
#22610=EDGE_LOOP ( 'NONE', ( #9041, #7900 ) ) ;
#22614=CARTESIAN_POINT ( 'NONE',  ( 282.6188186979285888, 272.3436892194421262, 145.4976310729378497 ) ) ;
#22629=DIRECTION ( 'NONE',  ( 0.000000000000000000, 0.000000000000000000, 1.000000000000000000 ) ) ;
#22632=DIRECTION ( 'NONE',  ( -0.000000000000000000, -0.000000000000000000, 1.000000000000000000 ) ) ;
#22636=DIRECTION ( 'NONE',  ( 0.000000000000000000, 0.000000000000000000, -1.000000000000000000 ) ) ;
#22645=AXIS2_PLACEMENT_3D ( 'NONE', #14366, #6974, #19755 ) ;
#22646=VERTEX_POINT ( 'NONE', #13484 ) ;
#22652=LINE ( 'NONE', #22419, #2631 ) ;
#22657=CARTESIAN_POINT ( 'NONE',  ( 280.7154581756738594, 271.5968359015654983, 148.5570580646227370 ) ) ;
#22667=FACE_OUTER_BOUND ( 'NONE', #5088, .T. ) ;
#22668=CARTESIAN_POINT ( 'NONE',  ( -7.703011046602857601E-15, -132.2000000000000455, 146.4928932188134638 ) ) ;
#22671=ORIENTED_EDGE ( 'NONE', *, *, #17978, .F. ) ;
#22675=AXIS2_PLACEMENT_3D ( 'NONE', #9550, #15126, #22455 ) ;
#22682=EDGE_LOOP ( 'NONE', ( #20002, #18571, #10999, #20625 ) ) ;
#22694=AXIS2_PLACEMENT_3D ( 'NONE', #8159, #23219, #13737 ) ;
#22699=EDGE_CURVE ( 'NONE', #19505, #6984, #9830, .T. ) ;
#22712=VECTOR ( 'NONE', #13721, 1000.000000000000000 ) ;
#22713=ORIENTED_EDGE ( 'NONE', *, *, #8610, .F. ) ;
#22722=DIRECTION ( 'NONE',  ( -0.000000000000000000, -0.000000000000000000, 1.000000000000000000 ) ) ;
#22723=EDGE_LOOP ( 'NONE', ( #9010, #5425, #4787, #8053 ) ) ;
#22724=CARTESIAN_POINT ( 'NONE',  ( 0.000000000000000000, 5.173457871231061435E-13, 150.2000000000009550 ) ) ;
#22730=CARTESIAN_POINT ( 'NONE',  ( -281.1021437883072736, 269.7094021484634254, 145.4974534559950712 ) ) ;
#22733=VECTOR ( 'NONE', #18585, 1000.000000000000000 ) ;
#22737=B_SPLINE_CURVE_WITH_KNOTS ( 'NONE', 3,
 ( #11942, #23232, #8389, #2726, #17457, #899, #15771, #6590, #19480, #6703, #1147, #15657, #22985, #13990, #4769, #5366 ),
 .UNSPECIFIED., .F., .F.,
 ( 4, 2, 2, 2, 2, 2, 2, 4 ),
 ( 0.000000000000000000, 0.0009361184303671995577, 0.001404177645550716991, 0.001872236860734234534, 0.002340296075917751642, 0.002808355291101269184, 0.003276414506284786726, 0.003744473721468304268 ),
 .UNSPECIFIED. ) ;
#22743=CARTESIAN_POINT ( 'NONE',  ( 282.1999999999999318, 268.0880230824753312, 146.3684665479256068 ) ) ;
#22749=EDGE_CURVE ( 'NONE', #22534, #9214, #21261, .T. ) ;
#22763=DIRECTION ( 'NONE',  ( -1.000000000000000000, 3.495664435217746987E-15, 0.000000000000000000 ) ) ;
#22770=DIRECTION ( 'NONE',  ( -1.000000000000000000, 0.000000000000000000, 0.000000000000000000 ) ) ;
#22791=CARTESIAN_POINT ( 'NONE',  ( 281.3681929792552410, 268.4822561791010571, 150.1663407402829762 ) ) ;
#22795=CARTESIAN_POINT ( 'NONE',  ( 282.1696999999999775, 267.7999999999999545, -146.4928932188133786 ) ) ;
#22806=FACE_OUTER_BOUND ( 'NONE', #23376, .T. ) ;
#22807=DIRECTION ( 'NONE',  ( 0.000000000000000000, -1.000000000000000000, -3.172065784643303781E-15 ) ) ;
#22817=DIRECTION ( 'NONE',  ( 0.000000000000000000, 0.000000000000000000, -1.000000000000000000 ) ) ;
#22818=DIRECTION ( 'NONE',  ( -1.000000000000000000, -0.000000000000000000, -0.000000000000000000 ) ) ;
#22828=ORIENTED_EDGE ( 'NONE', *, *, #4827, .F. ) ;
#22833=CARTESIAN_POINT ( 'NONE',  ( -281.3684637172360112, 268.4847249064868606, 150.2299999999999898 ) ) ;
#22842=VERTEX_POINT ( 'NONE', #16069 ) ;
#22844=ORIENTED_EDGE ( 'NONE', *, *, #18547, .T. ) ;
#22850=CARTESIAN_POINT ( 'NONE',  ( -280.0000000000000568, 269.9696999999999889, -144.9999999999999716 ) ) ;
#22860=ORIENTED_EDGE ( 'NONE', *, *, #22120, .F. ) ;
#22867=DIRECTION ( 'NONE',  ( 0.000000000000000000, 0.000000000000000000, 1.000000000000000000 ) ) ;
#22873=B_SPLINE_CURVE_WITH_KNOTS ( 'NONE', 3,
 ( #21598, #14254, #933, #23023, #15815, #2976, #23162, #12341, #6625, #19650, #8674, #3112, #17849, #5061, #12466, #6492 ),
 .UNSPECIFIED., .F., .F.,
 ( 4, 2, 2, 2, 2, 2, 2, 4 ),
 ( 2.775557561562891351E-17, 0.0009361184303670230496, 0.001404177645550584719, 0.001872236860734146496, 0.002340296075917707840, 0.002808355291101269618, 0.003276414506284831395, 0.003744473721468393173 ),
 .UNSPECIFIED. ) ;
#22886=CARTESIAN_POINT ( 'NONE',  ( -282.2000000000013529, -89.99999999999896261, -40.33333333333332860 ) ) ;
#22897=CARTESIAN_POINT ( 'NONE',  ( 280.5758453455903805, 269.9427398886703031, -145.2488155364688680 ) ) ;
#22901=CARTESIAN_POINT ( 'NONE',  ( -284.6728700860325603, 270.1062614524586252, 146.0570750465944343 ) ) ;
#22903=ORIENTED_EDGE ( 'NONE', *, *, #59, .T. ) ;
#22904=AXIS2_PLACEMENT_3D ( 'NONE', #14792, #15153, #9237 ) ;
#22905=EDGE_CURVE ( 'NONE', #21032, #3554, #11550, .T. ) ;
#22906=ORIENTED_EDGE ( 'NONE', *, *, #10634, .T. ) ;
#22908=LINE ( 'NONE', #6381, #12389 ) ;
#22918=VERTEX_POINT ( 'NONE', #21624 ) ;
#22919=VECTOR ( 'NONE', #244, 1000.000000000000000 ) ;
#22921=FACE_BOUND ( 'NONE', #20367, .T. ) ;
#22923=EDGE_LOOP ( 'NONE', ( #6628, #6128, #21829, #2796 ) ) ;
#22937=ORIENTED_EDGE ( 'NONE', *, *, #15455, .T. ) ;
#22944=AXIS2_PLACEMENT_3D ( 'NONE', #20996, #9905, #9533 ) ;
#22945=CARTESIAN_POINT ( 'NONE',  ( -280.2488155364689533, 269.9132285165672442, 145.5679143846943475 ) ) ;
#22950=PLANE ( 'NONE',  #8618 ) ;
#22956=ORIENTED_EDGE ( 'NONE', *, *, #3237, .T. ) ;
#22965=CARTESIAN_POINT ( 'NONE',  ( -281.4928932188134354, -129.2000000000000455, -152.4000000000012847 ) ) ;
#22966=DIRECTION ( 'NONE',  ( -0.000000000000000000, -0.000000000000000000, 1.000000000000000000 ) ) ;
#22967=CARTESIAN_POINT ( 'NONE',  ( -282.2000000000000455, 268.0880230824754449, -146.3684665479254932 ) ) ;
#22976=CARTESIAN_POINT ( 'NONE',  ( -282.2000000000012960, -74.99999999999899103, 90.00000000000000000 ) ) ;
#22980=CARTESIAN_POINT ( 'NONE',  ( -285.2000000000014666, -127.0000000000000568, 146.4928932188134638 ) ) ;
#22985=CARTESIAN_POINT ( 'NONE',  ( 280.5724317483737309, 269.9290760626066117, 145.2497115627124629 ) ) ;
#22987=LINE ( 'NONE', #8529, #13666 ) ;
#22988=VERTEX_POINT ( 'NONE', #16883 ) ;
#23017=AXIS2_PLACEMENT_3D ( 'NONE', #21000, #8445, #22807 ) ;
#23018=CARTESIAN_POINT ( 'NONE',  ( -282.2000000000013529, -89.99999999999896261, -42.98333333333330586 ) ) ;
#23023=CARTESIAN_POINT ( 'NONE',  ( 280.4357337430839721, 269.7771650631953548, 145.9755899421582512 ) ) ;
#23033=EDGE_CURVE ( 'NONE', #23104, #22426, #20256, .T. ) ;
#23036=VECTOR ( 'NONE', #21454, 1000.000000000000000 ) ;
#23046=CYLINDRICAL_SURFACE ( 'NONE', #17, 5.199999999999982414 ) ;
#23068=CARTESIAN_POINT ( 'NONE',  ( -280.1244266708878854, 269.9999999999999432, 145.2880230824751493 ) ) ;
#23076=AXIS2_PLACEMENT_3D ( 'NONE', #21579, #17833, #4680 ) ;
#23078=FACE_OUTER_BOUND ( 'NONE', #14802, .T. ) ;
#23079=ORIENTED_EDGE ( 'NONE', *, *, #10634, .F. ) ;
#23082=EDGE_LOOP ( 'NONE', ( #2516, #8766 ) ) ;
#23083=AXIS2_PLACEMENT_3D ( 'NONE', #9861, #13161, #9981 ) ;
#23087=VECTOR ( 'NONE', #23128, 1000.000000000000000 ) ;
#23096=CARTESIAN_POINT ( 'NONE',  ( -280.6807971656549512, 272.9999999999999432, -145.1244294735508618 ) ) ;
#23100=CARTESIAN_POINT ( 'NONE',  ( 99.99999999999997158, 34.99999999999995026, 150.2000000000010971 ) ) ;
#23104=VERTEX_POINT ( 'NONE', #697 ) ;
#23121=DIRECTION ( 'NONE',  ( 0.000000000000000000, 1.000000000000000000, -5.286776307738891306E-15 ) ) ;
#23122=VERTEX_POINT ( 'NONE', #23018 ) ;
#23128=DIRECTION ( 'NONE',  ( -1.000000000000000000, -0.000000000000000000, -0.000000000000000000 ) ) ;
#23138=AXIS2_PLACEMENT_3D ( 'NONE', #22298, #3942, #11352 ) ;
#23141=EDGE_CURVE ( 'NONE', #22099, #13958, #13116, .T. ) ;
#23146=EDGE_CURVE ( 'NONE', #1216, #17208, #13781, .T. ) ;
#23147=ORIENTED_EDGE ( 'NONE', *, *, #9299, .T. ) ;
#23149=DIRECTION ( 'NONE',  ( -0.000000000000000000, -1.000000000000000000, -0.000000000000000000 ) ) ;
#23158=AXIS2_PLACEMENT_3D ( 'NONE', #23211, #13843, #17320 ) ;
#23162=CARTESIAN_POINT ( 'NONE',  ( 280.6839617489739567, 269.4578961534455743, 146.4533442688711204 ) ) ;
#23166=CARTESIAN_POINT ( 'NONE',  ( -281.4928932188135491, 267.7999999999999545, 145.0000000000000284 ) ) ;
#23169=LINE ( 'NONE', #14029, #2112 ) ;
#23171=CARTESIAN_POINT ( 'NONE',  ( -287.4000000000014552, -132.2000000000000455, -146.4928932188134070 ) ) ;
#23182=CARTESIAN_POINT ( 'NONE',  ( -281.4928932188134922, -129.2000000000000455, -177.2000000000013529 ) ) ;
#23187=ADVANCED_FACE ( 'NONE', ( #22667 ), #21102, .T. ) ;
#23211=CARTESIAN_POINT ( 'NONE',  ( 45.00000000000000000, 272.9999999999999432, 0.000000000000000000 ) ) ;
#23212=EDGE_CURVE ( 'NONE', #3595, #13252, #7265, .T. ) ;
#23213=FACE_OUTER_BOUND ( 'NONE', #17289, .T. ) ;
#23215=CARTESIAN_POINT ( 'NONE',  ( -282.1132285165673466, 268.3679143846943020, -146.2440776823445390 ) ) ;
#23219=DIRECTION ( 'NONE',  ( -1.000000000000000000, 3.495664435217746987E-15, 0.000000000000000000 ) ) ;
#23221=ORIENTED_EDGE ( 'NONE', *, *, #19934, .T. ) ;
#23232=CARTESIAN_POINT ( 'NONE',  ( 282.1999999999998181, 268.0905802150184627, 146.3673618604587432 ) ) ;
#23244=DIRECTION ( 'NONE',  ( 1.000000000000000000, -3.495664435217746987E-15, -0.000000000000000000 ) ) ;
#23251=VECTOR ( 'NONE', #3064, 1000.000000000000000 ) ;
#23257=DIRECTION ( 'NONE',  ( 1.000000000000000000, -0.000000000000000000, -0.000000000000000000 ) ) ;
#23264=EDGE_LOOP ( 'NONE', ( #7739, #16918, #674, #22844 ) ) ;
#23270=ADVANCED_FACE ( 'NONE', ( #3460 ), #19643, .F. ) ;
#23272=B_SPLINE_CURVE_WITH_KNOTS ( 'NONE', 3,
 ( #8799, #6985, #21107, #15692, #6624, #14019, #21346, #13911, #10382, #19398, #19519, #2975, #1186, #8561, #15928, #4926 ),
 .UNSPECIFIED., .F., .F.,
 ( 4, 2, 2, 2, 2, 2, 2, 4 ),
 ( 0.000000000000000000, 0.0009361184303671104363, 0.001404177645550636760, 0.001872236860734162976, 0.002340296075917688758, 0.002808355291101215408, 0.003276414506284741190, 0.003744473721468266972 ),
 .UNSPECIFIED. ) ;
#23275=EDGE_CURVE ( 'NONE', #7513, #3739, #23736, .T. ) ;
#23286=ORIENTED_EDGE ( 'NONE', *, *, #21402, .F. ) ;
#23291=VECTOR ( 'NONE', #5397, 1000.000000000000000 ) ;
#23293=VECTOR ( 'NONE', #17492, 1000.000000000000000 ) ;
#23316=CARTESIAN_POINT ( 'NONE',  ( -280.6842353883612304, 269.4574776399286975, 146.4538215477170127 ) ) ;
#23317=EDGE_CURVE ( 'NONE', #18096, #22988, #11172, .T. ) ;
#23332=CARTESIAN_POINT ( 'NONE',  ( -280.5758453455904942, 269.9427398886703031, -145.2488155364688396 ) ) ;
#23335=EDGE_LOOP ( 'NONE', ( #5934, #23727, #17460, #14660 ) ) ;
#23343=CARTESIAN_POINT ( 'NONE',  ( 99.99999999999987210, -129.2000000000000455, 7.690461757479017101E-15 ) ) ;
#23359=ORIENTED_EDGE ( 'NONE', *, *, #13016, .F. ) ;
#23362=CARTESIAN_POINT ( 'NONE',  ( -285.2000000000008981, 30.00000000000101963, -105.0000000000000142 ) ) ;
#23373=CARTESIAN_POINT ( 'NONE',  ( -282.6054396500289840, 272.3132312761073308, -145.4975000228326394 ) ) ;
#23376=EDGE_LOOP ( 'NONE', ( #22828, #17881, #8927, #13784 ) ) ;
#23386=FACE_OUTER_BOUND ( 'NONE', #12289, .T. ) ;
#23390=CARTESIAN_POINT ( 'NONE',  ( -283.4314821058793541, 271.7107452280322377, 145.6845057130645102 ) ) ;
#23392=ORIENTED_EDGE ( 'NONE', *, *, #13203, .T. ) ;
#23394=AXIS2_PLACEMENT_3D ( 'NONE', #736, #15722, #12246 ) ;
#23401=CARTESIAN_POINT ( 'NONE',  ( 280.4976310729377360, 269.7223300543793698, 146.1079617568159961 ) ) ;
#23405=CIRCLE ( 'NONE', #12260, 2.649999999999971934 ) ;
#23409=ORIENTED_EDGE ( 'NONE', *, *, #11219, .F. ) ;
#23412=EDGE_CURVE ( 'NONE', #9258, #12339, #21937, .T. ) ;
#23414=CARTESIAN_POINT ( 'NONE',  ( -281.0570750465943775, 270.1062614524586820, -149.6728700860324750 ) ) ;
#23426=DIRECTION ( 'NONE',  ( 0.000000000000000000, 0.000000000000000000, 1.000000000000000000 ) ) ;
#23436=LINE ( 'NONE', #18014, #16146 ) ;
#23438=VECTOR ( 'NONE', #14421, 1000.000000000000000 ) ;
#23453=AXIS2_PLACEMENT_3D ( 'NONE', #17308, #6667, #756 ) ;
#23465=CARTESIAN_POINT ( 'NONE',  ( 0.000000000000000000, -132.2000000000000455, 7.703011046602857601E-15 ) ) ;
#23467=CARTESIAN_POINT ( 'NONE',  ( 99.99999999999987210, -129.2000000000000455, 177.2000000000014097 ) ) ;
#23473=AXIS2_PLACEMENT_3D ( 'NONE', #7799, #13393, #22636 ) ;
#23476=CARTESIAN_POINT ( 'NONE',  ( 99.99999999999987210, -132.2000000000001023, -113.4834095219707848 ) ) ;
#23479=AXIS2_PLACEMENT_3D ( 'NONE', #4922, #17721, #19880 ) ;
#23481=VECTOR ( 'NONE', #6069, 1000.000000000000000 ) ;
#23498=CARTESIAN_POINT ( 'NONE',  ( -281.4928932188135491, -127.0000000000000568, 152.4000000000014268 ) ) ;
#23501=VECTOR ( 'NONE', #19855, 1000.000000000000000 ) ;
#23505=AXIS2_PLACEMENT_3D ( 'NONE', #617, #17159, #18952 ) ;
#23530=EDGE_CURVE ( 'NONE', #7573, #18096, #4167, .T. ) ;
#23532=ADVANCED_FACE ( 'NONE', ( #12077 ), #4662, .F. ) ;
#23534=CARTESIAN_POINT ( 'NONE',  ( 280.2488155364687827, 272.8646579186752774, 146.3610889986682935 ) ) ;
#23540=AXIS2_PLACEMENT_3D ( 'NONE', #15553, #19610, #10482 ) ;
#23547=AXIS2_PLACEMENT_3D ( 'NONE', #8663, #13668, #1176 ) ;
#23549=DIRECTION ( 'NONE',  ( -1.000000000000000000, 3.495664435217746987E-15, 0.000000000000000000 ) ) ;
#23556=EDGE_CURVE ( 'NONE', #13791, #67, #3647, .T. ) ;
#23560=CYLINDRICAL_SURFACE ( 'NONE', #20642, 2.199999999999979750 ) ;
#23564=CARTESIAN_POINT ( 'NONE',  ( -288.2000000000008981, 35.00000000000100897, 107.6499999999999631 ) ) ;
#23565=CARTESIAN_POINT ( 'NONE',  ( -281.2447782964895282, 268.3743436287469422, 147.1433523009092994 ) ) ;
#23591=FACE_OUTER_BOUND ( 'NONE', #7541, .T. ) ;
#23603=CARTESIAN_POINT ( 'NONE',  ( -282.2000000000006708, 90.00000000000102318, -35.00000000000001421 ) ) ;
#23606=CARTESIAN_POINT ( 'NONE',  ( -281.3520027839448971, 269.5592670532759030, 145.6220388411722695 ) ) ;
#23615=CARTESIAN_POINT ( 'NONE',  ( 287.4000000000013415, -129.2000000000000455, 146.4928932188134638 ) ) ;
#23636=DIRECTION ( 'NONE',  ( 0.000000000000000000, -1.000000000000000000, 0.000000000000000000 ) ) ;
#23644=ORIENTED_EDGE ( 'NONE', *, *, #17526, .T. ) ;
#23648=ORIENTED_EDGE ( 'NONE', *, *, #8122, .F. ) ;
#23649=CARTESIAN_POINT ( 'NONE',  ( 282.6339272673396863, 272.3699028110927429, -145.4976310729377644 ) ) ;
#23665=EDGE_LOOP ( 'NONE', ( #22591, #15423, #18325, #2198 ) ) ;
#23670=FACE_OUTER_BOUND ( 'NONE', #2095, .T. ) ;
#23671=ADVANCED_FACE ( 'NONE', ( #13528 ), #672, .F. ) ;
#23676=ORIENTED_EDGE ( 'NONE', *, *, #10326, .F. ) ;
#23685=AXIS2_PLACEMENT_3D ( 'NONE', #17973, #16295, #23636 ) ;
#23686=EDGE_LOOP ( 'NONE', ( #23079, #17574, #4352, #9274 ) ) ;
#23688=CARTESIAN_POINT ( 'NONE',  ( -280.0000000000000568, 269.9999999999999432, -144.9999999999999716 ) ) ;
#23692=EDGE_CURVE ( 'NONE', #22099, #22022, #17564, .T. ) ;
#23713=ORIENTED_EDGE ( 'NONE', *, *, #3250, .F. ) ;
#23715=CARTESIAN_POINT ( 'NONE',  ( 280.6225751257470620, 269.5484459290826180, -146.3429506979392443 ) ) ;
#23719=FACE_OUTER_BOUND ( 'NONE', #6536, .T. ) ;
#23720=CARTESIAN_POINT ( 'NONE',  ( 280.6228333615949282, 271.9320353020573293, -148.1755088701071941 ) ) ;
#23727=ORIENTED_EDGE ( 'NONE', *, *, #18284, .F. ) ;
#23730=ADVANCED_FACE ( 'NONE', ( #18050 ), #4888, .F. ) ;
#23732=CARTESIAN_POINT ( 'NONE',  ( 7.703011046602857601E-15, -132.2000000000000455, -146.4928932188134070 ) ) ;
#23736=LINE ( 'NONE', #1534, #16538 ) ;
#23739=VERTEX_POINT ( 'NONE', #1497 ) ;
#23740=FACE_BOUND ( 'NONE', #16333, .T. ) ;
#23749=CARTESIAN_POINT ( 'NONE',  ( 280.6220388411721274, 269.5592670532759030, 146.3520027839448119 ) ) ;
#23757=DIRECTION ( 'NONE',  ( 1.000000000000000000, -3.495664435217746987E-15, -0.000000000000000000 ) ) ;
#23759=EDGE_LOOP ( 'NONE', ( #5475, #18939, #8937, #1330 ) ) ;
#23760=ORIENTED_EDGE ( 'NONE', *, *, #15372, .T. ) ;
#23764=CIRCLE ( 'NONE', #19922, 5.199999999999982414 ) ;
#23777=EDGE_CURVE ( 'NONE', #8918, #5697, #4611, .T. ) ;
#23778=ORIENTED_EDGE ( 'NONE', *, *, #9514, .T. ) ;
#23782=VERTEX_POINT ( 'NONE', #5022 ) ;
#23784=DIRECTION ( 'NONE',  ( -1.000000000000000000, 6.938893903907227392E-16, -2.425604463963772562E-30 ) ) ;
#23793=CARTESIAN_POINT ( 'NONE',  ( -285.2000000000014666, -127.0000000000000568, -146.4928932188134070 ) ) ;
#23794=AXIS2_PLACEMENT_3D ( 'NONE', #11266, #18808, #5800 ) ;
#23795=AXIS2_PLACEMENT_3D ( 'NONE', #20527, #7860, #20770 ) ;
#23801=ORIENTED_EDGE ( 'NONE', *, *, #2883, .T. ) ;
#23804=DIRECTION ( 'NONE',  ( -1.000000000000000000, -0.000000000000000000, -0.000000000000000000 ) ) ;
#23900=COLOUR_RGB('Light Blue',0.38,0.62,0.78);
#23901=FILL_AREA_STYLE_COLOUR('',#23900);
#23902=FILL_AREA_STYLE('',(#23901));
#23903=SURFACE_STYLE_FILL_AREA(#23902);
#23904=SURFACE_SIDE_STYLE('',(#23903));
#23905=SURFACE_STYLE_USAGE(.BOTH.,#23904);
#23906=PRESENTATION_STYLE_ASSIGNMENT((#23905));
ENDSEC;
END-ISO-10303-21;
